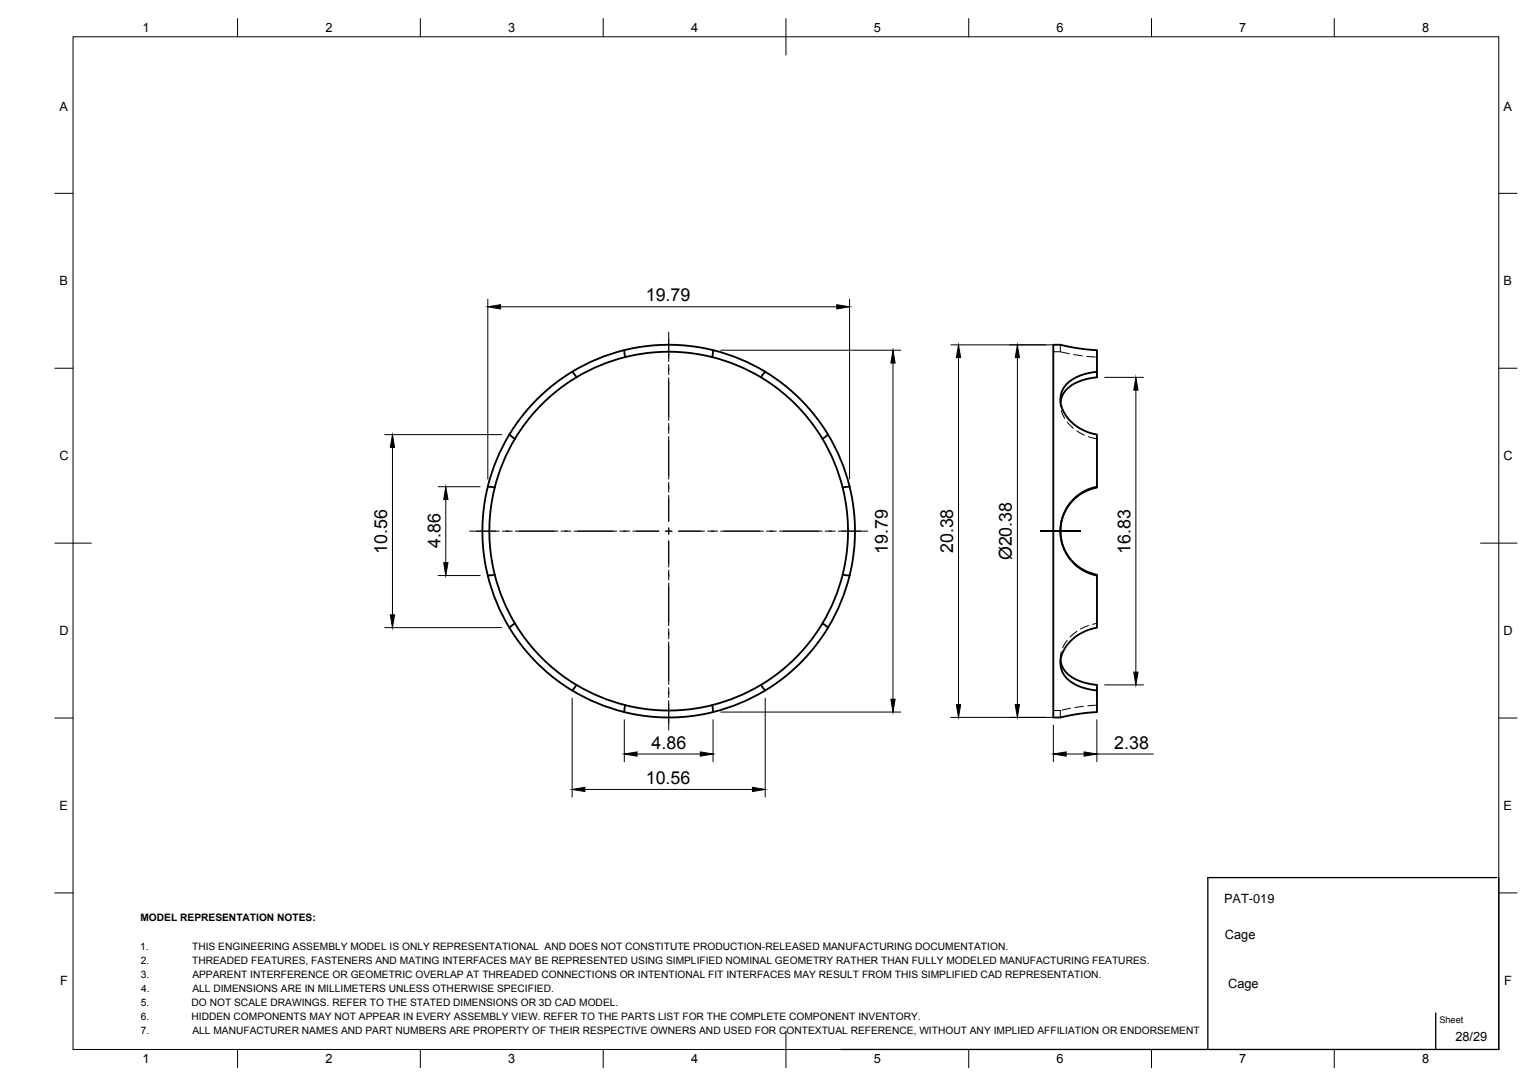
ISO-10303-21;
HEADER;
/* Generated by software containing ST-Developer
 * from STEP Tools, Inc. (www.steptools.com) 
 */

FILE_DESCRIPTION(
/* description */ ('Caster wheel assembly'),
/* implementation_level */ '2;1');

FILE_NAME(
/* name */ 'Cage.step',
/* time_stamp */ '2026-10-28T03:23:56-07:00',
/* author */ (''),
/* organization */ (''),
/* preprocessor_version */ 'ST-DEVELOPER v20.2',
/* originating_system */ 'Autodesk Translation Framework v15.17.0.0',
/* authorisation */ '');

FILE_SCHEMA (('AUTOMOTIVE_DESIGN { 1 0 10303 214 3 1 1 }'));
ENDSEC;

DATA;
#10=MECHANICAL_DESIGN_GEOMETRIC_PRESENTATION_REPRESENTATION('',(#249),#5385);
#11=B_SPLINE_CURVE_WITH_KNOTS('',3,(#4844,#4845,#4846,#4847,#4848,#4849,
#4850,#4851,#4852,#4853,#4854,#4855,#4856,#4857,#4858,#4859,#4860,#4861,
#4862,#4863,#4864,#4865),.UNSPECIFIED.,.F.,.F.,(4,2,2,2,2,2,2,2,2,2,4),
(0.0473477652366656,0.126350602536658,0.189525903804987,0.252701205073317,
0.313298422430275,0.373895639787233,0.434492857144191,0.495090074501149,
0.558265375769478,0.621440677037807,0.7004435143378),.UNSPECIFIED.);
#12=B_SPLINE_CURVE_WITH_KNOTS('',3,(#4869,#4870,#4871,#4872,#4873,#4874,
#4875,#4876,#4877,#4878,#4879,#4880,#4881,#4882,#4883,#4884,#4885,#4886,
#4887,#4888,#4889,#4890),.UNSPECIFIED.,.F.,.F.,(4,2,2,2,2,2,2,2,2,2,4),
(0.0464897534940957,0.0852567806515119,0.170513561303024,0.246687263103517,
0.308657850341199,0.370628437578881,0.432599024816563,0.494569612054245,
0.570743313854739,0.656000094506251,0.694767121663666),.UNSPECIFIED.);
#13=B_SPLINE_CURVE_WITH_KNOTS('',3,(#4896,#4897,#4898,#4899,#4900,#4901,
#4902,#4903,#4904,#4905,#4906,#4907,#4908,#4909,#4910,#4911,#4912,#4913,
#4914,#4915,#4916,#4917),.UNSPECIFIED.,.F.,.F.,(4,2,2,2,2,2,2,2,2,2,4),
(0.0464897534940957,0.0852567806515118,0.170513561303024,0.246687263103517,
0.308657850341199,0.370628437578881,0.432599024816563,0.494569612054245,
0.570743313854738,0.65600009450625,0.694767121663666),.UNSPECIFIED.);
#14=B_SPLINE_CURVE_WITH_KNOTS('',3,(#4921,#4922,#4923,#4924,#4925,#4926,
#4927,#4928,#4929,#4930,#4931,#4932,#4933,#4934,#4935,#4936,#4937,#4938,
#4939,#4940,#4941,#4942),.UNSPECIFIED.,.F.,.F.,(4,2,2,2,2,2,2,2,2,2,4),
(0.0464897534940957,0.0852567806515119,0.170513561303024,0.246687263103517,
0.308657850341199,0.370628437578881,0.432599024816563,0.494569612054245,
0.570743313854739,0.656000094506251,0.694767121663666),.UNSPECIFIED.);
#15=B_SPLINE_CURVE_WITH_KNOTS('',3,(#4946,#4947,#4948,#4949,#4950,#4951,
#4952,#4953,#4954,#4955,#4956,#4957),.UNSPECIFIED.,.F.,.F.,(4,2,2,2,2,4),
(0.0464897534940957,0.0852567806515119,0.170513561303024,0.246687263103517,
0.308657850341199,0.370628437578881),.UNSPECIFIED.);
#16=B_SPLINE_CURVE_WITH_KNOTS('',3,(#4962,#4963,#4964,#4965,#4966,#4967,
#4968,#4969,#4970,#4971,#4972,#4973),.UNSPECIFIED.,.F.,.F.,(4,2,2,2,2,4),
(0.370628437578881,0.432599024816563,0.494569612054245,0.570743313854738,
0.65600009450625,0.694767121663666),.UNSPECIFIED.);
#17=B_SPLINE_CURVE_WITH_KNOTS('',3,(#4977,#4978,#4979,#4980,#4981,#4982,
#4983,#4984,#4985,#4986,#4987,#4988,#4989,#4990,#4991,#4992,#4993,#4994,
#4995,#4996,#4997,#4998),.UNSPECIFIED.,.F.,.F.,(4,2,2,2,2,2,2,2,2,2,4),
(0.0464897534940957,0.0852567806515121,0.170513561303024,0.246687263103518,
0.308657850341199,0.370628437578881,0.432599024816563,0.494569612054245,
0.570743313854738,0.65600009450625,0.694767121663666),.UNSPECIFIED.);
#18=B_SPLINE_CURVE_WITH_KNOTS('',3,(#5002,#5003,#5004,#5005,#5006,#5007,
#5008,#5009,#5010,#5011,#5012,#5013,#5014,#5015,#5016,#5017,#5018,#5019,
#5020,#5021,#5022,#5023),.UNSPECIFIED.,.F.,.F.,(4,2,2,2,2,2,2,2,2,2,4),
(0.0464897534940957,0.0852567806515119,0.170513561303024,0.246687263103517,
0.308657850341199,0.370628437578881,0.432599024816563,0.494569612054245,
0.570743313854738,0.65600009450625,0.694767121663667),.UNSPECIFIED.);
#19=B_SPLINE_CURVE_WITH_KNOTS('',3,(#5027,#5028,#5029,#5030,#5031,#5032,
#5033,#5034,#5035,#5036,#5037,#5038,#5039,#5040,#5041,#5042,#5043,#5044,
#5045,#5046,#5047,#5048),.UNSPECIFIED.,.F.,.F.,(4,2,2,2,2,2,2,2,2,2,4),
(0.0464897534940957,0.0852567806515119,0.170513561303024,0.246687263103517,
0.308657850341199,0.370628437578881,0.432599024816563,0.494569612054245,
0.570743313854738,0.65600009450625,0.694767121663666),.UNSPECIFIED.);
#20=B_SPLINE_CURVE_WITH_KNOTS('',3,(#5052,#5053,#5054,#5055,#5056,#5057,
#5058,#5059,#5060,#5061,#5062,#5063,#5064,#5065,#5066,#5067,#5068,#5069,
#5070,#5071,#5072,#5073),.UNSPECIFIED.,.F.,.F.,(4,2,2,2,2,2,2,2,2,2,4),
(0.0464897534940957,0.0852567806515119,0.170513561303024,0.246687263103517,
0.308657850341199,0.370628437578881,0.432599024816563,0.494569612054245,
0.570743313854739,0.656000094506251,0.694767121663667),.UNSPECIFIED.);
#21=B_SPLINE_CURVE_WITH_KNOTS('',3,(#5081,#5082,#5083,#5084,#5085,#5086,
#5087,#5088,#5089,#5090,#5091,#5092,#5093,#5094,#5095,#5096,#5097,#5098,
#5099,#5100,#5101,#5102),.UNSPECIFIED.,.F.,.F.,(4,2,2,2,2,2,2,2,2,2,4),
(0.0473477652366656,0.126350602536658,0.189525903804987,0.252701205073316,
0.313298422430274,0.373895639787232,0.434492857144191,0.495090074501149,
0.558265375769478,0.621440677037807,0.7004435143378),.UNSPECIFIED.);
#22=B_SPLINE_CURVE_WITH_KNOTS('',3,(#5110,#5111,#5112,#5113,#5114,#5115,
#5116,#5117,#5118,#5119,#5120,#5121,#5122,#5123,#5124,#5125,#5126,#5127,
#5128,#5129,#5130,#5131),.UNSPECIFIED.,.F.,.F.,(4,2,2,2,2,2,2,2,2,2,4),
(0.0473477652366656,0.126350602536658,0.189525903804987,0.252701205073317,
0.313298422430275,0.373895639787233,0.434492857144191,0.495090074501149,
0.558265375769478,0.621440677037807,0.7004435143378),.UNSPECIFIED.);
#23=B_SPLINE_CURVE_WITH_KNOTS('',3,(#5140,#5141,#5142,#5143,#5144,#5145,
#5146,#5147,#5148,#5149,#5150,#5151),.UNSPECIFIED.,.F.,.F.,(4,2,2,2,2,4),
(0.0473477652366656,0.126350602536658,0.189525903804987,0.252701205073316,
0.313298422430275,0.373895639787233),.UNSPECIFIED.);
#24=B_SPLINE_CURVE_WITH_KNOTS('',3,(#5153,#5154,#5155,#5156,#5157,#5158,
#5159,#5160,#5161,#5162,#5163,#5164),.UNSPECIFIED.,.F.,.F.,(4,2,2,2,2,4),
(0.373895639787233,0.434492857144191,0.495090074501149,0.558265375769478,
0.621440677037807,0.7004435143378),.UNSPECIFIED.);
#25=B_SPLINE_CURVE_WITH_KNOTS('',3,(#5171,#5172,#5173,#5174,#5175,#5176,
#5177,#5178,#5179,#5180,#5181,#5182,#5183,#5184,#5185,#5186,#5187,#5188,
#5189,#5190,#5191,#5192),.UNSPECIFIED.,.F.,.F.,(4,2,2,2,2,2,2,2,2,2,4),
(0.0473477652366656,0.126350602536658,0.189525903804987,0.252701205073316,
0.313298422430275,0.373895639787233,0.434492857144191,0.495090074501149,
0.558265375769478,0.621440677037807,0.7004435143378),.UNSPECIFIED.);
#26=B_SPLINE_CURVE_WITH_KNOTS('',3,(#5200,#5201,#5202,#5203,#5204,#5205,
#5206,#5207,#5208,#5209,#5210,#5211,#5212,#5213,#5214,#5215,#5216,#5217,
#5218,#5219,#5220,#5221),.UNSPECIFIED.,.F.,.F.,(4,2,2,2,2,2,2,2,2,2,4),
(0.0473477652366656,0.126350602536658,0.189525903804987,0.252701205073317,
0.313298422430275,0.373895639787233,0.434492857144191,0.495090074501149,
0.558265375769478,0.621440677037807,0.7004435143378),.UNSPECIFIED.);
#27=B_SPLINE_CURVE_WITH_KNOTS('',3,(#5229,#5230,#5231,#5232,#5233,#5234,
#5235,#5236,#5237,#5238,#5239,#5240,#5241,#5242,#5243,#5244,#5245,#5246,
#5247,#5248,#5249,#5250),.UNSPECIFIED.,.F.,.F.,(4,2,2,2,2,2,2,2,2,2,4),
(0.0473477652366656,0.126350602536658,0.189525903804987,0.252701205073316,
0.313298422430275,0.373895639787233,0.434492857144191,0.495090074501149,
0.558265375769478,0.621440677037807,0.7004435143378),.UNSPECIFIED.);
#28=B_SPLINE_CURVE_WITH_KNOTS('',3,(#5259,#5260,#5261,#5262,#5263,#5264,
#5265,#5266,#5267,#5268,#5269,#5270,#5271,#5272,#5273,#5274,#5275,#5276,
#5277,#5278,#5279,#5280),.UNSPECIFIED.,.F.,.F.,(4,2,2,2,2,2,2,2,2,2,4),
(0.0473477652366656,0.126350602536658,0.189525903804987,0.252701205073317,
0.313298422430275,0.373895639787233,0.434492857144191,0.495090074501149,
0.558265375769478,0.621440677037807,0.7004435143378),.UNSPECIFIED.);
#37=SPHERICAL_SURFACE('',#3221,0.247676);
#38=SPHERICAL_SURFACE('',#3237,0.247676);
#39=SPHERICAL_SURFACE('',#3242,0.247676);
#40=SPHERICAL_SURFACE('',#3247,0.247676);
#41=SPHERICAL_SURFACE('',#3252,0.247676);
#42=SPHERICAL_SURFACE('',#3257,0.247676);
#43=SPHERICAL_SURFACE('',#3262,0.247676);
#44=SPHERICAL_SURFACE('',#3270,0.247676);
#198=SHAPE_REPRESENTATION_RELATIONSHIP('SRR','None',#5496,#220);
#220=ADVANCED_BREP_SHAPE_REPRESENTATION('',(#278),#5383);
#249=STYLED_ITEM('',(#5672),#278);
#278=MANIFOLD_SOLID_BREP('Continuous crown cage',#2677);
#328=FACE_BOUND('',#795,.T.);
#408=PLANE('',#3234);
#409=PLANE('',#3239);
#410=PLANE('',#3244);
#411=PLANE('',#3249);
#412=PLANE('',#3254);
#413=PLANE('',#3259);
#414=PLANE('',#3268);
#415=PLANE('',#3272);
#416=PLANE('',#3273);
#562=FACE_OUTER_BOUND('',#777,.T.);
#563=FACE_OUTER_BOUND('',#778,.T.);
#564=FACE_OUTER_BOUND('',#779,.T.);
#565=FACE_OUTER_BOUND('',#780,.T.);
#566=FACE_OUTER_BOUND('',#781,.T.);
#567=FACE_OUTER_BOUND('',#782,.T.);
#568=FACE_OUTER_BOUND('',#783,.T.);
#569=FACE_OUTER_BOUND('',#784,.T.);
#570=FACE_OUTER_BOUND('',#785,.T.);
#571=FACE_OUTER_BOUND('',#786,.T.);
#572=FACE_OUTER_BOUND('',#787,.T.);
#573=FACE_OUTER_BOUND('',#788,.T.);
#574=FACE_OUTER_BOUND('',#789,.T.);
#575=FACE_OUTER_BOUND('',#790,.T.);
#576=FACE_OUTER_BOUND('',#791,.T.);
#577=FACE_OUTER_BOUND('',#792,.T.);
#578=FACE_OUTER_BOUND('',#793,.T.);
#579=FACE_OUTER_BOUND('',#794,.T.);
#580=FACE_OUTER_BOUND('',#796,.T.);
#777=EDGE_LOOP('',(#2296,#2297,#2298,#2299));
#778=EDGE_LOOP('',(#2300,#2301,#2302,#2303,#2304,#2305,#2306,#2307,#2308,
#2309,#2310,#2311,#2312,#2313,#2314,#2315,#2316,#2317,#2318,#2319));
#779=EDGE_LOOP('',(#2320,#2321,#2322,#2323));
#780=EDGE_LOOP('',(#2324,#2325,#2326,#2327));
#781=EDGE_LOOP('',(#2328,#2329,#2330,#2331));
#782=EDGE_LOOP('',(#2332,#2333,#2334,#2335));
#783=EDGE_LOOP('',(#2336,#2337,#2338,#2339));
#784=EDGE_LOOP('',(#2340,#2341,#2342,#2343,#2344,#2345));
#785=EDGE_LOOP('',(#2346,#2347,#2348,#2349));
#786=EDGE_LOOP('',(#2350,#2351,#2352,#2353));
#787=EDGE_LOOP('',(#2354,#2355,#2356,#2357));
#788=EDGE_LOOP('',(#2358,#2359,#2360,#2361));
#789=EDGE_LOOP('',(#2362,#2363,#2364,#2365));
#790=EDGE_LOOP('',(#2366,#2367,#2368,#2369));
#791=EDGE_LOOP('',(#2370,#2371,#2372,#2373,#2374,#2375,#2376,#2377,#2378,
#2379,#2380,#2381,#2382,#2383,#2384,#2385,#2386,#2387,#2388,#2389));
#792=EDGE_LOOP('',(#2390,#2391,#2392,#2393));
#793=EDGE_LOOP('',(#2394,#2395,#2396,#2397));
#794=EDGE_LOOP('',(#2398));
#795=EDGE_LOOP('',(#2399));
#796=EDGE_LOOP('',(#2400,#2401,#2402,#2403));
#937=LINE('',#4959,#1071);
#938=LINE('',#5255,#1072);
#1071=VECTOR('',#4042,1.019052);
#1072=VECTOR('',#4119,0.980948);
#1194=CIRCLE('',#3222,0.243053047864041);
#1195=CIRCLE('',#3223,0.243053047864041);
#1196=CIRCLE('',#3225,1.019052);
#1197=CIRCLE('',#3226,1.019052);
#1198=CIRCLE('',#3227,1.019052);
#1199=CIRCLE('',#3228,1.019052);
#1200=CIRCLE('',#3229,1.019052);
#1201=CIRCLE('',#3230,1.019052);
#1202=CIRCLE('',#3231,1.019052);
#1203=CIRCLE('',#3232,1.019052);
#1204=CIRCLE('',#3233,1.019052);
#1205=CIRCLE('',#3235,0.980948);
#1206=CIRCLE('',#3236,0.243053047864041);
#1207=CIRCLE('',#3238,0.243053047864041);
#1208=CIRCLE('',#3240,0.980948);
#1209=CIRCLE('',#3241,0.243053047864041);
#1210=CIRCLE('',#3243,0.243053047864041);
#1211=CIRCLE('',#3245,0.980948);
#1212=CIRCLE('',#3246,0.243053047864041);
#1213=CIRCLE('',#3248,0.243053047864041);
#1214=CIRCLE('',#3250,0.980948);
#1215=CIRCLE('',#3251,0.243053047864041);
#1216=CIRCLE('',#3253,0.243053047864041);
#1217=CIRCLE('',#3255,0.980948);
#1218=CIRCLE('',#3256,0.243053047864041);
#1219=CIRCLE('',#3258,0.243053047864041);
#1220=CIRCLE('',#3260,0.980948);
#1221=CIRCLE('',#3261,0.243053047864041);
#1222=CIRCLE('',#3263,0.243053047864041);
#1223=CIRCLE('',#3265,0.980948);
#1224=CIRCLE('',#3266,0.980948);
#1225=CIRCLE('',#3267,0.980948);
#1226=CIRCLE('',#3269,0.243053047864041);
#1227=CIRCLE('',#3271,0.243053047864041);
#1415=VERTEX_POINT('',#4842);
#1416=VERTEX_POINT('',#4843);
#1417=VERTEX_POINT('',#4866);
#1418=VERTEX_POINT('',#4868);
#1419=VERTEX_POINT('',#4893);
#1420=VERTEX_POINT('',#4895);
#1421=VERTEX_POINT('',#4918);
#1422=VERTEX_POINT('',#4920);
#1423=VERTEX_POINT('',#4943);
#1424=VERTEX_POINT('',#4945);
#1425=VERTEX_POINT('',#4958);
#1426=VERTEX_POINT('',#4961);
#1427=VERTEX_POINT('',#4974);
#1428=VERTEX_POINT('',#4976);
#1429=VERTEX_POINT('',#4999);
#1430=VERTEX_POINT('',#5001);
#1431=VERTEX_POINT('',#5024);
#1432=VERTEX_POINT('',#5026);
#1433=VERTEX_POINT('',#5049);
#1434=VERTEX_POINT('',#5051);
#1435=VERTEX_POINT('',#5076);
#1436=VERTEX_POINT('',#5080);
#1437=VERTEX_POINT('',#5105);
#1438=VERTEX_POINT('',#5109);
#1439=VERTEX_POINT('',#5134);
#1440=VERTEX_POINT('',#5138);
#1441=VERTEX_POINT('',#5139);
#1442=VERTEX_POINT('',#5166);
#1443=VERTEX_POINT('',#5170);
#1444=VERTEX_POINT('',#5195);
#1445=VERTEX_POINT('',#5199);
#1446=VERTEX_POINT('',#5224);
#1447=VERTEX_POINT('',#5228);
#1448=VERTEX_POINT('',#5253);
#1449=VERTEX_POINT('',#5256);
#1450=VERTEX_POINT('',#5258);
#1716=EDGE_CURVE('',#1415,#1416,#11,.T.);
#1717=EDGE_CURVE('',#1417,#1415,#1194,.T.);
#1718=EDGE_CURVE('',#1418,#1417,#12,.T.);
#1719=EDGE_CURVE('',#1416,#1418,#1195,.T.);
#1720=EDGE_CURVE('',#1419,#1417,#1196,.T.);
#1721=EDGE_CURVE('',#1419,#1420,#13,.T.);
#1722=EDGE_CURVE('',#1421,#1420,#1197,.T.);
#1723=EDGE_CURVE('',#1421,#1422,#14,.T.);
#1724=EDGE_CURVE('',#1423,#1422,#1198,.T.);
#1725=EDGE_CURVE('',#1423,#1424,#15,.T.);
#1726=EDGE_CURVE('',#1424,#1425,#937,.T.);
#1727=EDGE_CURVE('',#1425,#1425,#1199,.T.);
#1728=EDGE_CURVE('',#1424,#1426,#16,.T.);
#1729=EDGE_CURVE('',#1427,#1426,#1200,.T.);
#1730=EDGE_CURVE('',#1427,#1428,#17,.T.);
#1731=EDGE_CURVE('',#1429,#1428,#1201,.T.);
#1732=EDGE_CURVE('',#1429,#1430,#18,.T.);
#1733=EDGE_CURVE('',#1431,#1430,#1202,.T.);
#1734=EDGE_CURVE('',#1431,#1432,#19,.T.);
#1735=EDGE_CURVE('',#1433,#1432,#1203,.T.);
#1736=EDGE_CURVE('',#1433,#1434,#20,.T.);
#1737=EDGE_CURVE('',#1418,#1434,#1204,.T.);
#1738=EDGE_CURVE('',#1415,#1435,#1205,.T.);
#1739=EDGE_CURVE('',#1435,#1419,#1206,.T.);
#1740=EDGE_CURVE('',#1436,#1435,#21,.T.);
#1741=EDGE_CURVE('',#1420,#1436,#1207,.T.);
#1742=EDGE_CURVE('',#1436,#1437,#1208,.T.);
#1743=EDGE_CURVE('',#1437,#1421,#1209,.T.);
#1744=EDGE_CURVE('',#1438,#1437,#22,.T.);
#1745=EDGE_CURVE('',#1422,#1438,#1210,.T.);
#1746=EDGE_CURVE('',#1438,#1439,#1211,.T.);
#1747=EDGE_CURVE('',#1439,#1423,#1212,.T.);
#1748=EDGE_CURVE('',#1440,#1441,#23,.T.);
#1749=EDGE_CURVE('',#1426,#1440,#1213,.T.);
#1750=EDGE_CURVE('',#1441,#1439,#24,.T.);
#1751=EDGE_CURVE('',#1440,#1442,#1214,.T.);
#1752=EDGE_CURVE('',#1442,#1427,#1215,.T.);
#1753=EDGE_CURVE('',#1443,#1442,#25,.T.);
#1754=EDGE_CURVE('',#1428,#1443,#1216,.T.);
#1755=EDGE_CURVE('',#1443,#1444,#1217,.T.);
#1756=EDGE_CURVE('',#1444,#1429,#1218,.T.);
#1757=EDGE_CURVE('',#1445,#1444,#26,.T.);
#1758=EDGE_CURVE('',#1430,#1445,#1219,.T.);
#1759=EDGE_CURVE('',#1445,#1446,#1220,.T.);
#1760=EDGE_CURVE('',#1446,#1431,#1221,.T.);
#1761=EDGE_CURVE('',#1447,#1446,#27,.T.);
#1762=EDGE_CURVE('',#1432,#1447,#1222,.T.);
#1763=EDGE_CURVE('',#1448,#1448,#1223,.T.);
#1764=EDGE_CURVE('',#1448,#1441,#938,.T.);
#1765=EDGE_CURVE('',#1449,#1416,#1224,.T.);
#1766=EDGE_CURVE('',#1449,#1450,#28,.T.);
#1767=EDGE_CURVE('',#1447,#1450,#1225,.T.);
#1768=EDGE_CURVE('',#1434,#1449,#1226,.T.);
#1769=EDGE_CURVE('',#1450,#1433,#1227,.T.);
#2296=ORIENTED_EDGE('',*,*,#1716,.F.);
#2297=ORIENTED_EDGE('',*,*,#1717,.F.);
#2298=ORIENTED_EDGE('',*,*,#1718,.F.);
#2299=ORIENTED_EDGE('',*,*,#1719,.F.);
#2300=ORIENTED_EDGE('',*,*,#1718,.T.);
#2301=ORIENTED_EDGE('',*,*,#1720,.F.);
#2302=ORIENTED_EDGE('',*,*,#1721,.T.);
#2303=ORIENTED_EDGE('',*,*,#1722,.F.);
#2304=ORIENTED_EDGE('',*,*,#1723,.T.);
#2305=ORIENTED_EDGE('',*,*,#1724,.F.);
#2306=ORIENTED_EDGE('',*,*,#1725,.T.);
#2307=ORIENTED_EDGE('',*,*,#1726,.T.);
#2308=ORIENTED_EDGE('',*,*,#1727,.F.);
#2309=ORIENTED_EDGE('',*,*,#1726,.F.);
#2310=ORIENTED_EDGE('',*,*,#1728,.T.);
#2311=ORIENTED_EDGE('',*,*,#1729,.F.);
#2312=ORIENTED_EDGE('',*,*,#1730,.T.);
#2313=ORIENTED_EDGE('',*,*,#1731,.F.);
#2314=ORIENTED_EDGE('',*,*,#1732,.T.);
#2315=ORIENTED_EDGE('',*,*,#1733,.F.);
#2316=ORIENTED_EDGE('',*,*,#1734,.T.);
#2317=ORIENTED_EDGE('',*,*,#1735,.F.);
#2318=ORIENTED_EDGE('',*,*,#1736,.T.);
#2319=ORIENTED_EDGE('',*,*,#1737,.F.);
#2320=ORIENTED_EDGE('',*,*,#1717,.T.);
#2321=ORIENTED_EDGE('',*,*,#1738,.T.);
#2322=ORIENTED_EDGE('',*,*,#1739,.T.);
#2323=ORIENTED_EDGE('',*,*,#1720,.T.);
#2324=ORIENTED_EDGE('',*,*,#1740,.F.);
#2325=ORIENTED_EDGE('',*,*,#1741,.F.);
#2326=ORIENTED_EDGE('',*,*,#1721,.F.);
#2327=ORIENTED_EDGE('',*,*,#1739,.F.);
#2328=ORIENTED_EDGE('',*,*,#1741,.T.);
#2329=ORIENTED_EDGE('',*,*,#1742,.T.);
#2330=ORIENTED_EDGE('',*,*,#1743,.T.);
#2331=ORIENTED_EDGE('',*,*,#1722,.T.);
#2332=ORIENTED_EDGE('',*,*,#1744,.F.);
#2333=ORIENTED_EDGE('',*,*,#1745,.F.);
#2334=ORIENTED_EDGE('',*,*,#1723,.F.);
#2335=ORIENTED_EDGE('',*,*,#1743,.F.);
#2336=ORIENTED_EDGE('',*,*,#1745,.T.);
#2337=ORIENTED_EDGE('',*,*,#1746,.T.);
#2338=ORIENTED_EDGE('',*,*,#1747,.T.);
#2339=ORIENTED_EDGE('',*,*,#1724,.T.);
#2340=ORIENTED_EDGE('',*,*,#1748,.F.);
#2341=ORIENTED_EDGE('',*,*,#1749,.F.);
#2342=ORIENTED_EDGE('',*,*,#1728,.F.);
#2343=ORIENTED_EDGE('',*,*,#1725,.F.);
#2344=ORIENTED_EDGE('',*,*,#1747,.F.);
#2345=ORIENTED_EDGE('',*,*,#1750,.F.);
#2346=ORIENTED_EDGE('',*,*,#1749,.T.);
#2347=ORIENTED_EDGE('',*,*,#1751,.T.);
#2348=ORIENTED_EDGE('',*,*,#1752,.T.);
#2349=ORIENTED_EDGE('',*,*,#1729,.T.);
#2350=ORIENTED_EDGE('',*,*,#1753,.F.);
#2351=ORIENTED_EDGE('',*,*,#1754,.F.);
#2352=ORIENTED_EDGE('',*,*,#1730,.F.);
#2353=ORIENTED_EDGE('',*,*,#1752,.F.);
#2354=ORIENTED_EDGE('',*,*,#1754,.T.);
#2355=ORIENTED_EDGE('',*,*,#1755,.T.);
#2356=ORIENTED_EDGE('',*,*,#1756,.T.);
#2357=ORIENTED_EDGE('',*,*,#1731,.T.);
#2358=ORIENTED_EDGE('',*,*,#1757,.F.);
#2359=ORIENTED_EDGE('',*,*,#1758,.F.);
#2360=ORIENTED_EDGE('',*,*,#1732,.F.);
#2361=ORIENTED_EDGE('',*,*,#1756,.F.);
#2362=ORIENTED_EDGE('',*,*,#1758,.T.);
#2363=ORIENTED_EDGE('',*,*,#1759,.T.);
#2364=ORIENTED_EDGE('',*,*,#1760,.T.);
#2365=ORIENTED_EDGE('',*,*,#1733,.T.);
#2366=ORIENTED_EDGE('',*,*,#1734,.F.);
#2367=ORIENTED_EDGE('',*,*,#1760,.F.);
#2368=ORIENTED_EDGE('',*,*,#1761,.F.);
#2369=ORIENTED_EDGE('',*,*,#1762,.F.);
#2370=ORIENTED_EDGE('',*,*,#1763,.F.);
#2371=ORIENTED_EDGE('',*,*,#1764,.T.);
#2372=ORIENTED_EDGE('',*,*,#1750,.T.);
#2373=ORIENTED_EDGE('',*,*,#1746,.F.);
#2374=ORIENTED_EDGE('',*,*,#1744,.T.);
#2375=ORIENTED_EDGE('',*,*,#1742,.F.);
#2376=ORIENTED_EDGE('',*,*,#1740,.T.);
#2377=ORIENTED_EDGE('',*,*,#1738,.F.);
#2378=ORIENTED_EDGE('',*,*,#1716,.T.);
#2379=ORIENTED_EDGE('',*,*,#1765,.F.);
#2380=ORIENTED_EDGE('',*,*,#1766,.T.);
#2381=ORIENTED_EDGE('',*,*,#1767,.F.);
#2382=ORIENTED_EDGE('',*,*,#1761,.T.);
#2383=ORIENTED_EDGE('',*,*,#1759,.F.);
#2384=ORIENTED_EDGE('',*,*,#1757,.T.);
#2385=ORIENTED_EDGE('',*,*,#1755,.F.);
#2386=ORIENTED_EDGE('',*,*,#1753,.T.);
#2387=ORIENTED_EDGE('',*,*,#1751,.F.);
#2388=ORIENTED_EDGE('',*,*,#1748,.T.);
#2389=ORIENTED_EDGE('',*,*,#1764,.F.);
#2390=ORIENTED_EDGE('',*,*,#1719,.T.);
#2391=ORIENTED_EDGE('',*,*,#1737,.T.);
#2392=ORIENTED_EDGE('',*,*,#1768,.T.);
#2393=ORIENTED_EDGE('',*,*,#1765,.T.);
#2394=ORIENTED_EDGE('',*,*,#1736,.F.);
#2395=ORIENTED_EDGE('',*,*,#1769,.F.);
#2396=ORIENTED_EDGE('',*,*,#1766,.F.);
#2397=ORIENTED_EDGE('',*,*,#1768,.F.);
#2398=ORIENTED_EDGE('',*,*,#1727,.T.);
#2399=ORIENTED_EDGE('',*,*,#1763,.T.);
#2400=ORIENTED_EDGE('',*,*,#1762,.T.);
#2401=ORIENTED_EDGE('',*,*,#1767,.T.);
#2402=ORIENTED_EDGE('',*,*,#1769,.T.);
#2403=ORIENTED_EDGE('',*,*,#1735,.T.);
#2475=CYLINDRICAL_SURFACE('',#3224,1.019052);
#2476=CYLINDRICAL_SURFACE('',#3264,0.980948);
#2622=ADVANCED_FACE('',(#562),#37,.F.);
#2623=ADVANCED_FACE('',(#563),#2475,.T.);
#2624=ADVANCED_FACE('',(#564),#408,.T.);
#2625=ADVANCED_FACE('',(#565),#38,.F.);
#2626=ADVANCED_FACE('',(#566),#409,.T.);
#2627=ADVANCED_FACE('',(#567),#39,.F.);
#2628=ADVANCED_FACE('',(#568),#410,.T.);
#2629=ADVANCED_FACE('',(#569),#40,.F.);
#2630=ADVANCED_FACE('',(#570),#411,.T.);
#2631=ADVANCED_FACE('',(#571),#41,.F.);
#2632=ADVANCED_FACE('',(#572),#412,.T.);
#2633=ADVANCED_FACE('',(#573),#42,.F.);
#2634=ADVANCED_FACE('',(#574),#413,.T.);
#2635=ADVANCED_FACE('',(#575),#43,.F.);
#2636=ADVANCED_FACE('',(#576),#2476,.F.);
#2637=ADVANCED_FACE('',(#577),#414,.T.);
#2638=ADVANCED_FACE('',(#578),#44,.F.);
#2639=ADVANCED_FACE('',(#579,#328),#415,.T.);
#2640=ADVANCED_FACE('',(#580),#416,.T.);
#2677=CLOSED_SHELL('',(#2622,#2623,#2624,#2625,#2626,#2627,#2628,#2629,
#2630,#2631,#2632,#2633,#2634,#2635,#2636,#2637,#2638,#2639,#2640));
#3220=AXIS2_PLACEMENT_3D('',#4840,#4026,#4027);
#3221=AXIS2_PLACEMENT_3D('',#4841,#4028,#4029);
#3222=AXIS2_PLACEMENT_3D('',#4867,#4030,#4031);
#3223=AXIS2_PLACEMENT_3D('',#4891,#4032,#4033);
#3224=AXIS2_PLACEMENT_3D('',#4892,#4034,#4035);
#3225=AXIS2_PLACEMENT_3D('',#4894,#4036,#4037);
#3226=AXIS2_PLACEMENT_3D('',#4919,#4038,#4039);
#3227=AXIS2_PLACEMENT_3D('',#4944,#4040,#4041);
#3228=AXIS2_PLACEMENT_3D('',#4960,#4043,#4044);
#3229=AXIS2_PLACEMENT_3D('',#4975,#4045,#4046);
#3230=AXIS2_PLACEMENT_3D('',#5000,#4047,#4048);
#3231=AXIS2_PLACEMENT_3D('',#5025,#4049,#4050);
#3232=AXIS2_PLACEMENT_3D('',#5050,#4051,#4052);
#3233=AXIS2_PLACEMENT_3D('',#5074,#4053,#4054);
#3234=AXIS2_PLACEMENT_3D('',#5075,#4055,#4056);
#3235=AXIS2_PLACEMENT_3D('',#5077,#4057,#4058);
#3236=AXIS2_PLACEMENT_3D('',#5078,#4059,#4060);
#3237=AXIS2_PLACEMENT_3D('',#5079,#4061,#4062);
#3238=AXIS2_PLACEMENT_3D('',#5103,#4063,#4064);
#3239=AXIS2_PLACEMENT_3D('',#5104,#4065,#4066);
#3240=AXIS2_PLACEMENT_3D('',#5106,#4067,#4068);
#3241=AXIS2_PLACEMENT_3D('',#5107,#4069,#4070);
#3242=AXIS2_PLACEMENT_3D('',#5108,#4071,#4072);
#3243=AXIS2_PLACEMENT_3D('',#5132,#4073,#4074);
#3244=AXIS2_PLACEMENT_3D('',#5133,#4075,#4076);
#3245=AXIS2_PLACEMENT_3D('',#5135,#4077,#4078);
#3246=AXIS2_PLACEMENT_3D('',#5136,#4079,#4080);
#3247=AXIS2_PLACEMENT_3D('',#5137,#4081,#4082);
#3248=AXIS2_PLACEMENT_3D('',#5152,#4083,#4084);
#3249=AXIS2_PLACEMENT_3D('',#5165,#4085,#4086);
#3250=AXIS2_PLACEMENT_3D('',#5167,#4087,#4088);
#3251=AXIS2_PLACEMENT_3D('',#5168,#4089,#4090);
#3252=AXIS2_PLACEMENT_3D('',#5169,#4091,#4092);
#3253=AXIS2_PLACEMENT_3D('',#5193,#4093,#4094);
#3254=AXIS2_PLACEMENT_3D('',#5194,#4095,#4096);
#3255=AXIS2_PLACEMENT_3D('',#5196,#4097,#4098);
#3256=AXIS2_PLACEMENT_3D('',#5197,#4099,#4100);
#3257=AXIS2_PLACEMENT_3D('',#5198,#4101,#4102);
#3258=AXIS2_PLACEMENT_3D('',#5222,#4103,#4104);
#3259=AXIS2_PLACEMENT_3D('',#5223,#4105,#4106);
#3260=AXIS2_PLACEMENT_3D('',#5225,#4107,#4108);
#3261=AXIS2_PLACEMENT_3D('',#5226,#4109,#4110);
#3262=AXIS2_PLACEMENT_3D('',#5227,#4111,#4112);
#3263=AXIS2_PLACEMENT_3D('',#5251,#4113,#4114);
#3264=AXIS2_PLACEMENT_3D('',#5252,#4115,#4116);
#3265=AXIS2_PLACEMENT_3D('',#5254,#4117,#4118);
#3266=AXIS2_PLACEMENT_3D('',#5257,#4120,#4121);
#3267=AXIS2_PLACEMENT_3D('',#5281,#4122,#4123);
#3268=AXIS2_PLACEMENT_3D('',#5282,#4124,#4125);
#3269=AXIS2_PLACEMENT_3D('',#5283,#4126,#4127);
#3270=AXIS2_PLACEMENT_3D('',#5284,#4128,#4129);
#3271=AXIS2_PLACEMENT_3D('',#5285,#4130,#4131);
#3272=AXIS2_PLACEMENT_3D('',#5286,#4132,#4133);
#3273=AXIS2_PLACEMENT_3D('',#5287,#4134,#4135);
#4026=DIRECTION('axis',(0.,0.,1.));
#4027=DIRECTION('refdir',(1.,0.,0.));
#4028=DIRECTION('center_axis',(0.,0.,1.));
#4029=DIRECTION('ref_axis',(1.,0.,0.));
#4030=DIRECTION('center_axis',(0.,-1.,0.));
#4031=DIRECTION('ref_axis',(0.,0.,-1.));
#4032=DIRECTION('center_axis',(0.,-1.,0.));
#4033=DIRECTION('ref_axis',(0.,0.,-1.));
#4034=DIRECTION('center_axis',(0.,1.,0.));
#4035=DIRECTION('ref_axis',(1.,0.,0.));
#4036=DIRECTION('center_axis',(0.,1.,0.));
#4037=DIRECTION('ref_axis',(1.,0.,0.));
#4038=DIRECTION('center_axis',(0.,1.,0.));
#4039=DIRECTION('ref_axis',(1.,0.,0.));
#4040=DIRECTION('center_axis',(0.,1.,0.));
#4041=DIRECTION('ref_axis',(1.,0.,0.));
#4042=DIRECTION('',(0.,-1.,0.));
#4043=DIRECTION('center_axis',(0.,-1.,0.));
#4044=DIRECTION('ref_axis',(1.,0.,0.));
#4045=DIRECTION('center_axis',(0.,1.,0.));
#4046=DIRECTION('ref_axis',(1.,0.,0.));
#4047=DIRECTION('center_axis',(0.,1.,0.));
#4048=DIRECTION('ref_axis',(1.,0.,0.));
#4049=DIRECTION('center_axis',(0.,1.,0.));
#4050=DIRECTION('ref_axis',(1.,0.,0.));
#4051=DIRECTION('center_axis',(0.,1.,0.));
#4052=DIRECTION('ref_axis',(1.,0.,0.));
#4053=DIRECTION('center_axis',(0.,1.,0.));
#4054=DIRECTION('ref_axis',(1.,0.,0.));
#4055=DIRECTION('center_axis',(0.,1.,0.));
#4056=DIRECTION('ref_axis',(1.,0.,0.));
#4057=DIRECTION('center_axis',(0.,-1.,0.));
#4058=DIRECTION('ref_axis',(1.,0.,0.));
#4059=DIRECTION('center_axis',(0.,-1.,0.));
#4060=DIRECTION('ref_axis',(0.,0.,-1.));
#4061=DIRECTION('center_axis',(6.12323399573677E-17,0.,1.));
#4062=DIRECTION('ref_axis',(1.,0.,0.));
#4063=DIRECTION('center_axis',(0.,-1.,0.));
#4064=DIRECTION('ref_axis',(0.,0.,-1.));
#4065=DIRECTION('center_axis',(0.,1.,0.));
#4066=DIRECTION('ref_axis',(1.,0.,0.));
#4067=DIRECTION('center_axis',(0.,-1.,0.));
#4068=DIRECTION('ref_axis',(1.,0.,0.));
#4069=DIRECTION('center_axis',(0.,-1.,0.));
#4070=DIRECTION('ref_axis',(0.,0.,-1.));
#4071=DIRECTION('center_axis',(0.,0.,1.));
#4072=DIRECTION('ref_axis',(1.,0.,0.));
#4073=DIRECTION('center_axis',(0.,-1.,0.));
#4074=DIRECTION('ref_axis',(0.,0.,-1.));
#4075=DIRECTION('center_axis',(0.,1.,0.));
#4076=DIRECTION('ref_axis',(1.,0.,0.));
#4077=DIRECTION('center_axis',(0.,-1.,0.));
#4078=DIRECTION('ref_axis',(1.,0.,0.));
#4079=DIRECTION('center_axis',(0.,-1.,0.));
#4080=DIRECTION('ref_axis',(0.,0.,-1.));
#4081=DIRECTION('center_axis',(0.,0.,1.));
#4082=DIRECTION('ref_axis',(1.,0.,0.));
#4083=DIRECTION('center_axis',(0.,-1.,0.));
#4084=DIRECTION('ref_axis',(0.,0.,-1.));
#4085=DIRECTION('center_axis',(0.,1.,0.));
#4086=DIRECTION('ref_axis',(1.,0.,0.));
#4087=DIRECTION('center_axis',(0.,-1.,0.));
#4088=DIRECTION('ref_axis',(1.,0.,0.));
#4089=DIRECTION('center_axis',(0.,-1.,0.));
#4090=DIRECTION('ref_axis',(0.,0.,-1.));
#4091=DIRECTION('center_axis',(0.,0.,1.));
#4092=DIRECTION('ref_axis',(1.,0.,0.));
#4093=DIRECTION('center_axis',(0.,-1.,0.));
#4094=DIRECTION('ref_axis',(0.,0.,-1.));
#4095=DIRECTION('center_axis',(0.,1.,0.));
#4096=DIRECTION('ref_axis',(1.,0.,0.));
#4097=DIRECTION('center_axis',(0.,-1.,0.));
#4098=DIRECTION('ref_axis',(1.,0.,0.));
#4099=DIRECTION('center_axis',(0.,-1.,0.));
#4100=DIRECTION('ref_axis',(0.,0.,-1.));
#4101=DIRECTION('center_axis',(6.12323399573676E-17,0.,1.));
#4102=DIRECTION('ref_axis',(1.,0.,0.));
#4103=DIRECTION('center_axis',(0.,-1.,0.));
#4104=DIRECTION('ref_axis',(0.,0.,-1.));
#4105=DIRECTION('center_axis',(0.,1.,0.));
#4106=DIRECTION('ref_axis',(1.,0.,0.));
#4107=DIRECTION('center_axis',(0.,-1.,0.));
#4108=DIRECTION('ref_axis',(1.,0.,0.));
#4109=DIRECTION('center_axis',(0.,-1.,0.));
#4110=DIRECTION('ref_axis',(0.,0.,-1.));
#4111=DIRECTION('center_axis',(0.,0.,1.));
#4112=DIRECTION('ref_axis',(1.,0.,0.));
#4113=DIRECTION('center_axis',(0.,-1.,0.));
#4114=DIRECTION('ref_axis',(0.,0.,-1.));
#4115=DIRECTION('center_axis',(0.,1.,0.));
#4116=DIRECTION('ref_axis',(1.,0.,0.));
#4117=DIRECTION('center_axis',(0.,1.,0.));
#4118=DIRECTION('ref_axis',(1.,0.,0.));
#4119=DIRECTION('',(0.,1.,0.));
#4120=DIRECTION('center_axis',(0.,-1.,0.));
#4121=DIRECTION('ref_axis',(1.,0.,0.));
#4122=DIRECTION('center_axis',(0.,-1.,0.));
#4123=DIRECTION('ref_axis',(1.,0.,0.));
#4124=DIRECTION('center_axis',(0.,1.,0.));
#4125=DIRECTION('ref_axis',(1.,0.,0.));
#4126=DIRECTION('center_axis',(0.,-1.,0.));
#4127=DIRECTION('ref_axis',(0.,0.,-1.));
#4128=DIRECTION('center_axis',(0.,0.,1.));
#4129=DIRECTION('ref_axis',(1.,0.,0.));
#4130=DIRECTION('center_axis',(0.,-1.,0.));
#4131=DIRECTION('ref_axis',(0.,0.,-1.));
#4132=DIRECTION('center_axis',(0.,-1.,0.));
#4133=DIRECTION('ref_axis',(-1.,0.,0.));
#4134=DIRECTION('center_axis',(0.,1.,0.));
#4135=DIRECTION('ref_axis',(1.,0.,0.));
#4840=CARTESIAN_POINT('',(0.,0.,0.));
#4841=CARTESIAN_POINT('Origin',(0.707106781186547,0.,0.707106781186548));
#4842=CARTESIAN_POINT('',(0.504455939115715,-0.04763,0.841298510752802));
#4843=CARTESIAN_POINT('',(0.841298510752802,-0.04763,0.504455939115715));
#4844=CARTESIAN_POINT('Ctrl Pts',(0.504455939115715,-0.04763,0.841298510752802));
#4845=CARTESIAN_POINT('Ctrl Pts',(0.508899795931835,-0.0740444353928835,
0.838633903678357));
#4846=CARTESIAN_POINT('Ctrl Pts',(0.517157748491652,-0.0999305678883309,
0.833661031856294));
#4847=CARTESIAN_POINT('Ctrl Pts',(0.537715343527944,-0.142345102874864,
0.820511285096538));
#4848=CARTESIAN_POINT('Ctrl Pts',(0.548874290046456,-0.159766064500479,
0.813159949759));
#4849=CARTESIAN_POINT('Ctrl Pts',(0.573915184558107,-0.190326085855194,
0.795684265985089));
#4850=CARTESIAN_POINT('Ctrl Pts',(0.587792702767295,-0.203463743702801,
0.78555112003688));
#4851=CARTESIAN_POINT('Ctrl Pts',(0.615966552324775,-0.224161999508995,
0.763642258217233));
#4852=CARTESIAN_POINT('Ctrl Pts',(0.631684198665438,-0.232861760990032,
0.750785745543687));
#4853=CARTESIAN_POINT('Ctrl Pts',(0.663382628119203,-0.244251601209411,
0.722929908501543));
#4854=CARTESIAN_POINT('Ctrl Pts',(0.679352081686668,-0.246942143572133,
0.707917883896095));
#4855=CARTESIAN_POINT('Ctrl Pts',(0.707917883896095,-0.246942143572133,
0.679352081686668));
#4856=CARTESIAN_POINT('Ctrl Pts',(0.722929908501543,-0.244251601209411,
0.663382628119203));
#4857=CARTESIAN_POINT('Ctrl Pts',(0.750785745543687,-0.232861760990032,
0.631684198665439));
#4858=CARTESIAN_POINT('Ctrl Pts',(0.763642258217232,-0.224161999508995,
0.615966552324775));
#4859=CARTESIAN_POINT('Ctrl Pts',(0.78555112003688,-0.203463743702801,0.587792702767295));
#4860=CARTESIAN_POINT('Ctrl Pts',(0.795684265985088,-0.190326085855194,
0.573915184558108));
#4861=CARTESIAN_POINT('Ctrl Pts',(0.813159949759,-0.15976606450048,0.548874290046456));
#4862=CARTESIAN_POINT('Ctrl Pts',(0.820511285096538,-0.142345102874864,
0.537715343527944));
#4863=CARTESIAN_POINT('Ctrl Pts',(0.833661031856294,-0.099930567888331,
0.517157748491653));
#4864=CARTESIAN_POINT('Ctrl Pts',(0.838633903678357,-0.0740444353928835,
0.508899795931835));
#4865=CARTESIAN_POINT('Ctrl Pts',(0.841298510752801,-0.0476299999999999,
0.504455939115715));
#4866=CARTESIAN_POINT('',(0.528110872004958,-0.04763,0.871530771444223));
#4867=CARTESIAN_POINT('Origin',(0.707106781186547,-0.04763,0.707106781186548));
#4868=CARTESIAN_POINT('',(0.871530771444223,-0.04763,0.528110872004959));
#4869=CARTESIAN_POINT('Ctrl Pts',(0.871530771444223,-0.0476300000000001,
0.528110872004958));
#4870=CARTESIAN_POINT('Ctrl Pts',(0.87014664509073,-0.0609922781173483,
0.530395067942936));
#4871=CARTESIAN_POINT('Ctrl Pts',(0.868149331745851,-0.0742967091364493,
0.533674141594226));
#4872=CARTESIAN_POINT('Ctrl Pts',(0.85981294420286,-0.115492077056649,0.54708917182331));
#4873=CARTESIAN_POINT('Ctrl Pts',(0.850993704737257,-0.141695629206859,
0.560922177770136));
#4874=CARTESIAN_POINT('Ctrl Pts',(0.830754510485543,-0.181890537957859,
0.590422647829571));
#4875=CARTESIAN_POINT('Ctrl Pts',(0.816896541396381,-0.201072148666545,
0.609616703125488));
#4876=CARTESIAN_POINT('Ctrl Pts',(0.792310597819928,-0.223955109275652,
0.641117951819998));
#4877=CARTESIAN_POINT('Ctrl Pts',(0.779109323683612,-0.232742381310829,
0.657208095763053));
#4878=CARTESIAN_POINT('Ctrl Pts',(0.750552691816206,-0.244234834628584,
0.68964083160521));
#4879=CARTESIAN_POINT('Ctrl Pts',(0.735185187071673,-0.246942143572133,
0.705971972091755));
#4880=CARTESIAN_POINT('Ctrl Pts',(0.705971972091754,-0.246942143572133,
0.735185187071673));
#4881=CARTESIAN_POINT('Ctrl Pts',(0.689640831605209,-0.244234834628584,
0.750552691816206));
#4882=CARTESIAN_POINT('Ctrl Pts',(0.657208095763052,-0.232742381310829,
0.779109323683612));
#4883=CARTESIAN_POINT('Ctrl Pts',(0.641117951819998,-0.223955109275652,
0.792310597819928));
#4884=CARTESIAN_POINT('Ctrl Pts',(0.609616703125487,-0.201072148666545,
0.816896541396382));
#4885=CARTESIAN_POINT('Ctrl Pts',(0.590422647829571,-0.181890537957858,
0.830754510485544));
#4886=CARTESIAN_POINT('Ctrl Pts',(0.560922177770135,-0.141695629206858,
0.850993704737257));
#4887=CARTESIAN_POINT('Ctrl Pts',(0.547089171823309,-0.115492077056649,
0.859812944202861));
#4888=CARTESIAN_POINT('Ctrl Pts',(0.533674141594226,-0.0742967091364491,
0.868149331745852));
#4889=CARTESIAN_POINT('Ctrl Pts',(0.530395067942936,-0.0609922781173483,
0.870146645090731));
#4890=CARTESIAN_POINT('Ctrl Pts',(0.528110872004958,-0.0476300000000001,
0.871530771444223));
#4891=CARTESIAN_POINT('Origin',(0.707106781186547,-0.04763,0.707106781186548));
#4892=CARTESIAN_POINT('Origin',(0.,-0.166705,0.));
#4893=CARTESIAN_POINT('',(0.242834539687906,-0.04763,0.989696097314));
#4894=CARTESIAN_POINT('Origin',(0.,-0.04763,0.));
#4895=CARTESIAN_POINT('',(-0.242834539687907,-0.04763,0.989696097314));
#4896=CARTESIAN_POINT('Ctrl Pts',(0.242834539687906,-0.04763,0.989696097314));
#4897=CARTESIAN_POINT('Ctrl Pts',(0.24024064412003,-0.0609922781173483,
0.990332542620729));
#4898=CARTESIAN_POINT('Ctrl Pts',(0.236509675094874,-0.0742967091364492,
0.991238884025248));
#4899=CARTESIAN_POINT('Ctrl Pts',(0.221129100087819,-0.115492077056649,
0.994830026707808));
#4900=CARTESIAN_POINT('Ctrl Pts',(0.205111543747588,-0.141695629206859,
0.998375294985966));
#4901=CARTESIAN_POINT('Ctrl Pts',(0.169940289819232,-0.181890537957859,
1.00492400591205));
#4902=CARTESIAN_POINT('Ctrl Pts',(0.1465689792446,-0.201072148666545,1.00869718865384));
#4903=CARTESIAN_POINT('Ctrl Pts',(0.106909345252087,-0.223955109275652,
1.01358704779679));
#4904=CARTESIAN_POINT('Ctrl Pts',(0.0861971848975941,-0.232742381310829,
1.0156297872271));
#4905=CARTESIAN_POINT('Ctrl Pts',(0.0430711894098822,-0.244234834628584,
1.01837060663223));
#4906=CARTESIAN_POINT('Ctrl Pts',(0.0206568624125605,-0.246942143572133,
1.019052));
#4907=CARTESIAN_POINT('Ctrl Pts',(-0.0206568624125608,-0.246942143572133,
1.019052));
#4908=CARTESIAN_POINT('Ctrl Pts',(-0.0430711894098825,-0.244234834628584,
1.01837060663223));
#4909=CARTESIAN_POINT('Ctrl Pts',(-0.0861971848975943,-0.232742381310829,
1.0156297872271));
#4910=CARTESIAN_POINT('Ctrl Pts',(-0.106909345252088,-0.223955109275652,
1.01358704779679));
#4911=CARTESIAN_POINT('Ctrl Pts',(-0.1465689792446,-0.201072148666545,1.00869718865384));
#4912=CARTESIAN_POINT('Ctrl Pts',(-0.169940289819232,-0.181890537957859,
1.00492400591205));
#4913=CARTESIAN_POINT('Ctrl Pts',(-0.205111543747588,-0.141695629206859,
0.998375294985966));
#4914=CARTESIAN_POINT('Ctrl Pts',(-0.221129100087819,-0.115492077056649,
0.994830026707808));
#4915=CARTESIAN_POINT('Ctrl Pts',(-0.236509675094875,-0.0742967091364493,
0.991238884025248));
#4916=CARTESIAN_POINT('Ctrl Pts',(-0.24024064412003,-0.0609922781173483,
0.990332542620729));
#4917=CARTESIAN_POINT('Ctrl Pts',(-0.242834539687907,-0.04763,0.989696097314));
#4918=CARTESIAN_POINT('',(-0.528110872004959,-0.04763,0.871530771444223));
#4919=CARTESIAN_POINT('Origin',(0.,-0.04763,0.));
#4920=CARTESIAN_POINT('',(-0.871530771444223,-0.04763,0.528110872004958));
#4921=CARTESIAN_POINT('Ctrl Pts',(-0.528110872004958,-0.0476300000000001,
0.871530771444223));
#4922=CARTESIAN_POINT('Ctrl Pts',(-0.530395067942936,-0.0609922781173484,
0.87014664509073));
#4923=CARTESIAN_POINT('Ctrl Pts',(-0.533674141594226,-0.0742967091364493,
0.868149331745851));
#4924=CARTESIAN_POINT('Ctrl Pts',(-0.54708917182331,-0.115492077056649,
0.85981294420286));
#4925=CARTESIAN_POINT('Ctrl Pts',(-0.560922177770136,-0.141695629206859,
0.850993704737257));
#4926=CARTESIAN_POINT('Ctrl Pts',(-0.590422647829571,-0.181890537957859,
0.830754510485543));
#4927=CARTESIAN_POINT('Ctrl Pts',(-0.609616703125488,-0.201072148666545,
0.816896541396381));
#4928=CARTESIAN_POINT('Ctrl Pts',(-0.641117951819998,-0.223955109275652,
0.792310597819928));
#4929=CARTESIAN_POINT('Ctrl Pts',(-0.657208095763053,-0.232742381310829,
0.779109323683611));
#4930=CARTESIAN_POINT('Ctrl Pts',(-0.68964083160521,-0.244234834628584,
0.750552691816205));
#4931=CARTESIAN_POINT('Ctrl Pts',(-0.705971972091755,-0.246942143572133,
0.735185187071673));
#4932=CARTESIAN_POINT('Ctrl Pts',(-0.735185187071673,-0.246942143572133,
0.705971972091754));
#4933=CARTESIAN_POINT('Ctrl Pts',(-0.750552691816206,-0.244234834628584,
0.689640831605209));
#4934=CARTESIAN_POINT('Ctrl Pts',(-0.779109323683612,-0.232742381310829,
0.657208095763052));
#4935=CARTESIAN_POINT('Ctrl Pts',(-0.792310597819928,-0.223955109275652,
0.641117951819998));
#4936=CARTESIAN_POINT('Ctrl Pts',(-0.816896541396382,-0.201072148666545,
0.609616703125487));
#4937=CARTESIAN_POINT('Ctrl Pts',(-0.830754510485544,-0.181890537957858,
0.590422647829571));
#4938=CARTESIAN_POINT('Ctrl Pts',(-0.850993704737257,-0.141695629206858,
0.560922177770135));
#4939=CARTESIAN_POINT('Ctrl Pts',(-0.859812944202861,-0.115492077056649,
0.547089171823309));
#4940=CARTESIAN_POINT('Ctrl Pts',(-0.868149331745852,-0.0742967091364491,
0.533674141594226));
#4941=CARTESIAN_POINT('Ctrl Pts',(-0.870146645090731,-0.0609922781173483,
0.530395067942936));
#4942=CARTESIAN_POINT('Ctrl Pts',(-0.871530771444223,-0.04763,0.528110872004958));
#4943=CARTESIAN_POINT('',(-0.989696097314,-0.04763,0.242834539687906));
#4944=CARTESIAN_POINT('Origin',(0.,-0.04763,0.));
#4945=CARTESIAN_POINT('',(-1.019052,-0.246942143572133,1.248489836334E-16));
#4946=CARTESIAN_POINT('Ctrl Pts',(-0.989696097314,-0.04763,0.242834539687906));
#4947=CARTESIAN_POINT('Ctrl Pts',(-0.990332542620729,-0.0609922781173483,
0.24024064412003));
#4948=CARTESIAN_POINT('Ctrl Pts',(-0.991238884025248,-0.0742967091364492,
0.236509675094874));
#4949=CARTESIAN_POINT('Ctrl Pts',(-0.994830026707808,-0.115492077056649,
0.221129100087819));
#4950=CARTESIAN_POINT('Ctrl Pts',(-0.998375294985966,-0.141695629206859,
0.205111543747588));
#4951=CARTESIAN_POINT('Ctrl Pts',(-1.00492400591205,-0.181890537957859,
0.169940289819232));
#4952=CARTESIAN_POINT('Ctrl Pts',(-1.00869718865384,-0.201072148666545,
0.1465689792446));
#4953=CARTESIAN_POINT('Ctrl Pts',(-1.01358704779679,-0.223955109275652,
0.106909345252088));
#4954=CARTESIAN_POINT('Ctrl Pts',(-1.0156297872271,-0.232742381310829,0.0861971848975944));
#4955=CARTESIAN_POINT('Ctrl Pts',(-1.01837060663223,-0.244234834628584,
0.0430711894098825));
#4956=CARTESIAN_POINT('Ctrl Pts',(-1.019052,-0.246942143572133,0.0206568624125608));
#4957=CARTESIAN_POINT('Ctrl Pts',(-1.019052,-0.246942143572133,1.2490009027033E-16));
#4958=CARTESIAN_POINT('',(-1.019052,-0.28578,1.24797876996471E-16));
#4959=CARTESIAN_POINT('',(-1.019052,-0.166705,1.24797876996471E-16));
#4960=CARTESIAN_POINT('Origin',(0.,-0.28578,0.));
#4961=CARTESIAN_POINT('',(-0.989696097314,-0.04763,-0.242834539687906));
#4962=CARTESIAN_POINT('Ctrl Pts',(-1.019052,-0.246942143572133,1.2490009027033E-16));
#4963=CARTESIAN_POINT('Ctrl Pts',(-1.019052,-0.246942143572133,-0.0206568624125605));
#4964=CARTESIAN_POINT('Ctrl Pts',(-1.01837060663223,-0.244234834628584,
-0.0430711894098822));
#4965=CARTESIAN_POINT('Ctrl Pts',(-1.0156297872271,-0.232742381310829,-0.0861971848975941));
#4966=CARTESIAN_POINT('Ctrl Pts',(-1.01358704779679,-0.223955109275652,
-0.106909345252087));
#4967=CARTESIAN_POINT('Ctrl Pts',(-1.00869718865384,-0.201072148666546,
-0.1465689792446));
#4968=CARTESIAN_POINT('Ctrl Pts',(-1.00492400591205,-0.181890537957859,
-0.169940289819232));
#4969=CARTESIAN_POINT('Ctrl Pts',(-0.998375294985966,-0.141695629206859,
-0.205111543747588));
#4970=CARTESIAN_POINT('Ctrl Pts',(-0.994830026707808,-0.11549207705665,
-0.221129100087819));
#4971=CARTESIAN_POINT('Ctrl Pts',(-0.991238884025248,-0.0742967091364495,
-0.236509675094874));
#4972=CARTESIAN_POINT('Ctrl Pts',(-0.990332542620729,-0.0609922781173484,
-0.24024064412003));
#4973=CARTESIAN_POINT('Ctrl Pts',(-0.989696097314,-0.0476300000000001,-0.242834539687907));
#4974=CARTESIAN_POINT('',(-0.871530771444223,-0.04763,-0.528110872004958));
#4975=CARTESIAN_POINT('Origin',(0.,-0.04763,0.));
#4976=CARTESIAN_POINT('',(-0.528110872004958,-0.04763,-0.871530771444223));
#4977=CARTESIAN_POINT('Ctrl Pts',(-0.871530771444223,-0.0476300000000001,
-0.528110872004958));
#4978=CARTESIAN_POINT('Ctrl Pts',(-0.87014664509073,-0.0609922781173484,
-0.530395067942936));
#4979=CARTESIAN_POINT('Ctrl Pts',(-0.868149331745851,-0.0742967091364494,
-0.533674141594226));
#4980=CARTESIAN_POINT('Ctrl Pts',(-0.85981294420286,-0.115492077056649,
-0.54708917182331));
#4981=CARTESIAN_POINT('Ctrl Pts',(-0.850993704737257,-0.141695629206859,
-0.560922177770136));
#4982=CARTESIAN_POINT('Ctrl Pts',(-0.830754510485543,-0.181890537957859,
-0.590422647829571));
#4983=CARTESIAN_POINT('Ctrl Pts',(-0.816896541396381,-0.201072148666546,
-0.609616703125488));
#4984=CARTESIAN_POINT('Ctrl Pts',(-0.792310597819928,-0.223955109275652,
-0.641117951819999));
#4985=CARTESIAN_POINT('Ctrl Pts',(-0.779109323683611,-0.232742381310829,
-0.657208095763053));
#4986=CARTESIAN_POINT('Ctrl Pts',(-0.750552691816205,-0.244234834628584,
-0.68964083160521));
#4987=CARTESIAN_POINT('Ctrl Pts',(-0.735185187071673,-0.246942143572133,
-0.705971972091755));
#4988=CARTESIAN_POINT('Ctrl Pts',(-0.705971972091754,-0.246942143572133,
-0.735185187071673));
#4989=CARTESIAN_POINT('Ctrl Pts',(-0.68964083160521,-0.244234834628584,
-0.750552691816206));
#4990=CARTESIAN_POINT('Ctrl Pts',(-0.657208095763052,-0.232742381310829,
-0.779109323683612));
#4991=CARTESIAN_POINT('Ctrl Pts',(-0.641117951819998,-0.223955109275652,
-0.792310597819928));
#4992=CARTESIAN_POINT('Ctrl Pts',(-0.609616703125488,-0.201072148666545,
-0.816896541396381));
#4993=CARTESIAN_POINT('Ctrl Pts',(-0.590422647829571,-0.181890537957859,
-0.830754510485543));
#4994=CARTESIAN_POINT('Ctrl Pts',(-0.560922177770136,-0.141695629206859,
-0.850993704737257));
#4995=CARTESIAN_POINT('Ctrl Pts',(-0.54708917182331,-0.115492077056649,
-0.85981294420286));
#4996=CARTESIAN_POINT('Ctrl Pts',(-0.533674141594226,-0.0742967091364494,
-0.868149331745852));
#4997=CARTESIAN_POINT('Ctrl Pts',(-0.530395067942936,-0.0609922781173484,
-0.870146645090731));
#4998=CARTESIAN_POINT('Ctrl Pts',(-0.528110872004958,-0.0476300000000001,
-0.871530771444223));
#4999=CARTESIAN_POINT('',(-0.242834539687906,-0.04763,-0.989696097314));
#5000=CARTESIAN_POINT('Origin',(0.,-0.04763,0.));
#5001=CARTESIAN_POINT('',(0.242834539687906,-0.04763,-0.989696097314));
#5002=CARTESIAN_POINT('Ctrl Pts',(-0.242834539687907,-0.04763,-0.989696097314));
#5003=CARTESIAN_POINT('Ctrl Pts',(-0.24024064412003,-0.0609922781173483,
-0.990332542620729));
#5004=CARTESIAN_POINT('Ctrl Pts',(-0.236509675094874,-0.0742967091364493,
-0.991238884025248));
#5005=CARTESIAN_POINT('Ctrl Pts',(-0.221129100087819,-0.115492077056649,
-0.994830026707808));
#5006=CARTESIAN_POINT('Ctrl Pts',(-0.205111543747588,-0.141695629206859,
-0.998375294985966));
#5007=CARTESIAN_POINT('Ctrl Pts',(-0.169940289819232,-0.181890537957859,
-1.00492400591205));
#5008=CARTESIAN_POINT('Ctrl Pts',(-0.1465689792446,-0.201072148666545,-1.00869718865384));
#5009=CARTESIAN_POINT('Ctrl Pts',(-0.106909345252087,-0.223955109275652,
-1.01358704779679));
#5010=CARTESIAN_POINT('Ctrl Pts',(-0.0861971848975942,-0.232742381310829,
-1.0156297872271));
#5011=CARTESIAN_POINT('Ctrl Pts',(-0.0430711894098823,-0.244234834628584,
-1.01837060663223));
#5012=CARTESIAN_POINT('Ctrl Pts',(-0.0206568624125606,-0.246942143572133,
-1.019052));
#5013=CARTESIAN_POINT('Ctrl Pts',(0.0206568624125607,-0.246942143572133,
-1.019052));
#5014=CARTESIAN_POINT('Ctrl Pts',(0.0430711894098824,-0.244234834628584,
-1.01837060663223));
#5015=CARTESIAN_POINT('Ctrl Pts',(0.0861971848975943,-0.232742381310829,
-1.0156297872271));
#5016=CARTESIAN_POINT('Ctrl Pts',(0.106909345252088,-0.223955109275652,
-1.01358704779679));
#5017=CARTESIAN_POINT('Ctrl Pts',(0.1465689792446,-0.201072148666545,-1.00869718865384));
#5018=CARTESIAN_POINT('Ctrl Pts',(0.169940289819232,-0.181890537957859,
-1.00492400591205));
#5019=CARTESIAN_POINT('Ctrl Pts',(0.205111543747588,-0.141695629206859,
-0.998375294985966));
#5020=CARTESIAN_POINT('Ctrl Pts',(0.221129100087819,-0.115492077056649,
-0.994830026707808));
#5021=CARTESIAN_POINT('Ctrl Pts',(0.236509675094874,-0.0742967091364493,
-0.991238884025248));
#5022=CARTESIAN_POINT('Ctrl Pts',(0.24024064412003,-0.0609922781173484,
-0.990332542620729));
#5023=CARTESIAN_POINT('Ctrl Pts',(0.242834539687907,-0.04763,-0.989696097314));
#5024=CARTESIAN_POINT('',(0.528110872004958,-0.04763,-0.871530771444223));
#5025=CARTESIAN_POINT('Origin',(0.,-0.04763,0.));
#5026=CARTESIAN_POINT('',(0.871530771444223,-0.04763,-0.528110872004958));
#5027=CARTESIAN_POINT('Ctrl Pts',(0.528110872004958,-0.0476300000000001,
-0.871530771444223));
#5028=CARTESIAN_POINT('Ctrl Pts',(0.530395067942936,-0.0609922781173484,
-0.870146645090731));
#5029=CARTESIAN_POINT('Ctrl Pts',(0.533674141594226,-0.0742967091364493,
-0.868149331745851));
#5030=CARTESIAN_POINT('Ctrl Pts',(0.54708917182331,-0.115492077056649,-0.85981294420286));
#5031=CARTESIAN_POINT('Ctrl Pts',(0.560922177770136,-0.141695629206859,
-0.850993704737257));
#5032=CARTESIAN_POINT('Ctrl Pts',(0.590422647829571,-0.181890537957859,
-0.830754510485543));
#5033=CARTESIAN_POINT('Ctrl Pts',(0.609616703125488,-0.201072148666545,
-0.816896541396381));
#5034=CARTESIAN_POINT('Ctrl Pts',(0.641117951819998,-0.223955109275652,
-0.792310597819928));
#5035=CARTESIAN_POINT('Ctrl Pts',(0.657208095763053,-0.232742381310829,
-0.779109323683612));
#5036=CARTESIAN_POINT('Ctrl Pts',(0.68964083160521,-0.244234834628584,-0.750552691816206));
#5037=CARTESIAN_POINT('Ctrl Pts',(0.705971972091755,-0.246942143572133,
-0.735185187071673));
#5038=CARTESIAN_POINT('Ctrl Pts',(0.735185187071673,-0.246942143572133,
-0.705971972091754));
#5039=CARTESIAN_POINT('Ctrl Pts',(0.750552691816206,-0.244234834628584,
-0.68964083160521));
#5040=CARTESIAN_POINT('Ctrl Pts',(0.779109323683612,-0.232742381310829,
-0.657208095763053));
#5041=CARTESIAN_POINT('Ctrl Pts',(0.792310597819928,-0.223955109275652,
-0.641117951819998));
#5042=CARTESIAN_POINT('Ctrl Pts',(0.816896541396381,-0.201072148666545,
-0.609616703125488));
#5043=CARTESIAN_POINT('Ctrl Pts',(0.830754510485543,-0.181890537957859,
-0.590422647829571));
#5044=CARTESIAN_POINT('Ctrl Pts',(0.850993704737257,-0.141695629206859,
-0.560922177770136));
#5045=CARTESIAN_POINT('Ctrl Pts',(0.85981294420286,-0.115492077056649,-0.54708917182331));
#5046=CARTESIAN_POINT('Ctrl Pts',(0.868149331745851,-0.0742967091364493,
-0.533674141594226));
#5047=CARTESIAN_POINT('Ctrl Pts',(0.870146645090731,-0.0609922781173484,
-0.530395067942936));
#5048=CARTESIAN_POINT('Ctrl Pts',(0.871530771444223,-0.0476300000000001,
-0.528110872004958));
#5049=CARTESIAN_POINT('',(0.989696097314,-0.04763,-0.242834539687906));
#5050=CARTESIAN_POINT('Origin',(0.,-0.04763,0.));
#5051=CARTESIAN_POINT('',(0.989696097314,-0.04763,0.242834539687906));
#5052=CARTESIAN_POINT('Ctrl Pts',(0.989696097314,-0.04763,-0.242834539687907));
#5053=CARTESIAN_POINT('Ctrl Pts',(0.990332542620729,-0.0609922781173483,
-0.24024064412003));
#5054=CARTESIAN_POINT('Ctrl Pts',(0.991238884025248,-0.0742967091364493,
-0.236509675094874));
#5055=CARTESIAN_POINT('Ctrl Pts',(0.994830026707808,-0.115492077056649,
-0.221129100087819));
#5056=CARTESIAN_POINT('Ctrl Pts',(0.998375294985966,-0.141695629206859,
-0.205111543747588));
#5057=CARTESIAN_POINT('Ctrl Pts',(1.00492400591205,-0.181890537957859,-0.169940289819232));
#5058=CARTESIAN_POINT('Ctrl Pts',(1.00869718865384,-0.201072148666545,-0.1465689792446));
#5059=CARTESIAN_POINT('Ctrl Pts',(1.01358704779679,-0.223955109275652,-0.106909345252087));
#5060=CARTESIAN_POINT('Ctrl Pts',(1.0156297872271,-0.232742381310829,-0.0861971848975942));
#5061=CARTESIAN_POINT('Ctrl Pts',(1.01837060663223,-0.244234834628584,-0.0430711894098823));
#5062=CARTESIAN_POINT('Ctrl Pts',(1.019052,-0.246942143572133,-0.0206568624125607));
#5063=CARTESIAN_POINT('Ctrl Pts',(1.019052,-0.246942143572133,0.0206568624125607));
#5064=CARTESIAN_POINT('Ctrl Pts',(1.01837060663223,-0.244234834628584,0.0430711894098823));
#5065=CARTESIAN_POINT('Ctrl Pts',(1.0156297872271,-0.232742381310829,0.0861971848975942));
#5066=CARTESIAN_POINT('Ctrl Pts',(1.01358704779679,-0.223955109275652,0.106909345252087));
#5067=CARTESIAN_POINT('Ctrl Pts',(1.00869718865384,-0.201072148666545,0.1465689792446));
#5068=CARTESIAN_POINT('Ctrl Pts',(1.00492400591205,-0.181890537957859,0.169940289819232));
#5069=CARTESIAN_POINT('Ctrl Pts',(0.998375294985966,-0.141695629206859,
0.205111543747588));
#5070=CARTESIAN_POINT('Ctrl Pts',(0.994830026707808,-0.115492077056649,
0.221129100087819));
#5071=CARTESIAN_POINT('Ctrl Pts',(0.991238884025248,-0.0742967091364492,
0.236509675094874));
#5072=CARTESIAN_POINT('Ctrl Pts',(0.990332542620729,-0.0609922781173483,
0.24024064412003));
#5073=CARTESIAN_POINT('Ctrl Pts',(0.989696097314,-0.04763,0.242834539687907));
#5074=CARTESIAN_POINT('Origin',(0.,-0.04763,0.));
#5075=CARTESIAN_POINT('Origin',(0.,-0.04763,0.));
#5076=CARTESIAN_POINT('',(0.238183666596899,-0.04763,0.951592097314));
#5077=CARTESIAN_POINT('Origin',(0.,-0.04763,0.));
#5078=CARTESIAN_POINT('Origin',(-1.94289029309402E-16,-0.04763,1.));
#5079=CARTESIAN_POINT('Origin',(-1.94289029309402E-16,0.,1.));
#5080=CARTESIAN_POINT('',(-0.2381836665969,-0.04763,0.951592097314));
#5081=CARTESIAN_POINT('Ctrl Pts',(-0.238183666596899,-0.0476299999999999,
0.951592097314));
#5082=CARTESIAN_POINT('Ctrl Pts',(-0.233157223576062,-0.0740444353928835,
0.952850216871763));
#5083=CARTESIAN_POINT('Ctrl Pts',(-0.223801617934946,-0.0999305678883309,
0.955173119738174));
#5084=CARTESIAN_POINT('Ctrl Pts',(-0.199966927975188,-0.142345102874864,
0.960411259488514));
#5085=CARTESIAN_POINT('Ctrl Pts',(-0.1868781821531,-0.159766064500479,0.963103647174702));
#5086=CARTESIAN_POINT('Ctrl Pts',(-0.15681442133453,-0.190326085855194,
0.968453058988463));
#5087=CARTESIAN_POINT('Ctrl Pts',(-0.139836317888043,-0.203463743702801,
0.971100730005489));
#5088=CARTESIAN_POINT('Ctrl Pts',(-0.104422493053067,-0.224161999508995,
0.975530745318961));
#5089=CARTESIAN_POINT('Ctrl Pts',(-0.0842175114474176,-0.232861760990032,
0.977553872336861));
#5090=CARTESIAN_POINT('Ctrl Pts',(-0.0421062857595701,-0.244251601209411,
0.980270995488453));
#5091=CARTESIAN_POINT('Ctrl Pts',(-0.0201990724523197,-0.246942143572133,
0.980948));
#5092=CARTESIAN_POINT('Ctrl Pts',(0.020199072452319,-0.246942143572133,
0.980948));
#5093=CARTESIAN_POINT('Ctrl Pts',(0.0421062857595694,-0.244251601209411,
0.980270995488454));
#5094=CARTESIAN_POINT('Ctrl Pts',(0.0842175114474169,-0.232861760990032,
0.977553872336861));
#5095=CARTESIAN_POINT('Ctrl Pts',(0.104422493053067,-0.224161999508995,
0.975530745318961));
#5096=CARTESIAN_POINT('Ctrl Pts',(0.139836317888042,-0.203463743702801,
0.971100730005489));
#5097=CARTESIAN_POINT('Ctrl Pts',(0.15681442133453,-0.190326085855194,0.968453058988463));
#5098=CARTESIAN_POINT('Ctrl Pts',(0.1868781821531,-0.15976606450048,0.963103647174702));
#5099=CARTESIAN_POINT('Ctrl Pts',(0.199966927975188,-0.142345102874864,
0.960411259488514));
#5100=CARTESIAN_POINT('Ctrl Pts',(0.223801617934945,-0.0999305678883309,
0.955173119738174));
#5101=CARTESIAN_POINT('Ctrl Pts',(0.233157223576061,-0.0740444353928835,
0.952850216871763));
#5102=CARTESIAN_POINT('Ctrl Pts',(0.238183666596899,-0.0476299999999999,
0.951592097314));
#5103=CARTESIAN_POINT('Origin',(-1.94289029309402E-16,-0.04763,1.));
#5104=CARTESIAN_POINT('Origin',(0.,-0.04763,0.));
#5105=CARTESIAN_POINT('',(-0.504455939115715,-0.04763,0.841298510752802));
#5106=CARTESIAN_POINT('Origin',(0.,-0.04763,0.));
#5107=CARTESIAN_POINT('Origin',(-0.707106781186548,-0.04763,0.707106781186547));
#5108=CARTESIAN_POINT('Origin',(-0.707106781186548,0.,0.707106781186547));
#5109=CARTESIAN_POINT('',(-0.841298510752802,-0.04763,0.504455939115715));
#5110=CARTESIAN_POINT('Ctrl Pts',(-0.841298510752802,-0.04763,0.504455939115715));
#5111=CARTESIAN_POINT('Ctrl Pts',(-0.838633903678357,-0.0740444353928835,
0.508899795931835));
#5112=CARTESIAN_POINT('Ctrl Pts',(-0.833661031856294,-0.0999305678883309,
0.517157748491652));
#5113=CARTESIAN_POINT('Ctrl Pts',(-0.820511285096538,-0.142345102874864,
0.537715343527944));
#5114=CARTESIAN_POINT('Ctrl Pts',(-0.813159949759,-0.159766064500479,0.548874290046456));
#5115=CARTESIAN_POINT('Ctrl Pts',(-0.795684265985089,-0.190326085855194,
0.573915184558107));
#5116=CARTESIAN_POINT('Ctrl Pts',(-0.78555112003688,-0.203463743702801,
0.587792702767295));
#5117=CARTESIAN_POINT('Ctrl Pts',(-0.763642258217233,-0.224161999508995,
0.615966552324775));
#5118=CARTESIAN_POINT('Ctrl Pts',(-0.750785745543687,-0.232861760990032,
0.631684198665438));
#5119=CARTESIAN_POINT('Ctrl Pts',(-0.722929908501543,-0.244251601209411,
0.663382628119203));
#5120=CARTESIAN_POINT('Ctrl Pts',(-0.707917883896095,-0.246942143572133,
0.679352081686668));
#5121=CARTESIAN_POINT('Ctrl Pts',(-0.679352081686668,-0.246942143572133,
0.707917883896095));
#5122=CARTESIAN_POINT('Ctrl Pts',(-0.663382628119203,-0.244251601209411,
0.722929908501544));
#5123=CARTESIAN_POINT('Ctrl Pts',(-0.631684198665438,-0.232861760990031,
0.750785745543687));
#5124=CARTESIAN_POINT('Ctrl Pts',(-0.615966552324775,-0.224161999508995,
0.763642258217233));
#5125=CARTESIAN_POINT('Ctrl Pts',(-0.587792702767295,-0.203463743702801,
0.78555112003688));
#5126=CARTESIAN_POINT('Ctrl Pts',(-0.573915184558107,-0.190326085855194,
0.795684265985088));
#5127=CARTESIAN_POINT('Ctrl Pts',(-0.548874290046456,-0.159766064500479,
0.813159949759));
#5128=CARTESIAN_POINT('Ctrl Pts',(-0.537715343527944,-0.142345102874864,
0.820511285096538));
#5129=CARTESIAN_POINT('Ctrl Pts',(-0.517157748491652,-0.0999305678883309,
0.833661031856294));
#5130=CARTESIAN_POINT('Ctrl Pts',(-0.508899795931835,-0.0740444353928835,
0.838633903678357));
#5131=CARTESIAN_POINT('Ctrl Pts',(-0.504455939115716,-0.04763,0.841298510752801));
#5132=CARTESIAN_POINT('Origin',(-0.707106781186548,-0.04763,0.707106781186547));
#5133=CARTESIAN_POINT('Origin',(0.,-0.04763,0.));
#5134=CARTESIAN_POINT('',(-0.951592097314,-0.04763,0.238183666596899));
#5135=CARTESIAN_POINT('Origin',(0.,-0.04763,0.));
#5136=CARTESIAN_POINT('Origin',(-1.,-0.04763,-1.11022302462516E-16));
#5137=CARTESIAN_POINT('Origin',(-1.,0.,-1.11022302462516E-16));
#5138=CARTESIAN_POINT('',(-0.951592097314,-0.04763,-0.2381836665969));
#5139=CARTESIAN_POINT('',(-0.980948,-0.246942143572133,1.08514323328844E-18));
#5140=CARTESIAN_POINT('Ctrl Pts',(-0.951592097314,-0.04763,-0.238183666596899));
#5141=CARTESIAN_POINT('Ctrl Pts',(-0.952850216871763,-0.0740444353928835,
-0.233157223576062));
#5142=CARTESIAN_POINT('Ctrl Pts',(-0.955173119738174,-0.0999305678883309,
-0.223801617934946));
#5143=CARTESIAN_POINT('Ctrl Pts',(-0.960411259488514,-0.142345102874864,
-0.199966927975188));
#5144=CARTESIAN_POINT('Ctrl Pts',(-0.963103647174702,-0.159766064500479,
-0.1868781821531));
#5145=CARTESIAN_POINT('Ctrl Pts',(-0.968453058988463,-0.190326085855194,
-0.15681442133453));
#5146=CARTESIAN_POINT('Ctrl Pts',(-0.971100730005489,-0.203463743702801,
-0.139836317888043));
#5147=CARTESIAN_POINT('Ctrl Pts',(-0.975530745318961,-0.224161999508995,
-0.104422493053067));
#5148=CARTESIAN_POINT('Ctrl Pts',(-0.977553872336861,-0.232861760990032,
-0.0842175114474175));
#5149=CARTESIAN_POINT('Ctrl Pts',(-0.980270995488453,-0.244251601209411,
-0.0421062857595699));
#5150=CARTESIAN_POINT('Ctrl Pts',(-0.980948,-0.246942143572133,-0.0201990724523195));
#5151=CARTESIAN_POINT('Ctrl Pts',(-0.980948,-0.246942143572133,-1.17961196366423E-16));
#5152=CARTESIAN_POINT('Origin',(-1.,-0.04763,-1.11022302462516E-16));
#5153=CARTESIAN_POINT('Ctrl Pts',(-0.980948,-0.246942143572133,-1.17961196366423E-16));
#5154=CARTESIAN_POINT('Ctrl Pts',(-0.980948,-0.246942143572133,0.0201990724523192));
#5155=CARTESIAN_POINT('Ctrl Pts',(-0.980270995488453,-0.244251601209411,
0.0421062857595695));
#5156=CARTESIAN_POINT('Ctrl Pts',(-0.977553872336861,-0.232861760990032,
0.0842175114474169));
#5157=CARTESIAN_POINT('Ctrl Pts',(-0.975530745318961,-0.224161999508995,
0.104422493053066));
#5158=CARTESIAN_POINT('Ctrl Pts',(-0.971100730005489,-0.203463743702801,
0.139836317888042));
#5159=CARTESIAN_POINT('Ctrl Pts',(-0.968453058988463,-0.190326085855194,
0.15681442133453));
#5160=CARTESIAN_POINT('Ctrl Pts',(-0.963103647174702,-0.15976606450048,
0.1868781821531));
#5161=CARTESIAN_POINT('Ctrl Pts',(-0.960411259488514,-0.142345102874864,
0.199966927975188));
#5162=CARTESIAN_POINT('Ctrl Pts',(-0.955173119738174,-0.099930567888331,
0.223801617934945));
#5163=CARTESIAN_POINT('Ctrl Pts',(-0.952850216871763,-0.0740444353928835,
0.233157223576061));
#5164=CARTESIAN_POINT('Ctrl Pts',(-0.951592097314,-0.04763,0.238183666596899));
#5165=CARTESIAN_POINT('Origin',(0.,-0.04763,0.));
#5166=CARTESIAN_POINT('',(-0.841298510752802,-0.04763,-0.504455939115715));
#5167=CARTESIAN_POINT('Origin',(0.,-0.04763,0.));
#5168=CARTESIAN_POINT('Origin',(-0.707106781186547,-0.04763,-0.707106781186548));
#5169=CARTESIAN_POINT('Origin',(-0.707106781186547,0.,-0.707106781186548));
#5170=CARTESIAN_POINT('',(-0.504455939115715,-0.04763,-0.841298510752802));
#5171=CARTESIAN_POINT('Ctrl Pts',(-0.504455939115715,-0.04763,-0.841298510752802));
#5172=CARTESIAN_POINT('Ctrl Pts',(-0.508899795931835,-0.0740444353928835,
-0.838633903678357));
#5173=CARTESIAN_POINT('Ctrl Pts',(-0.517157748491652,-0.0999305678883309,
-0.833661031856294));
#5174=CARTESIAN_POINT('Ctrl Pts',(-0.537715343527944,-0.142345102874864,
-0.820511285096538));
#5175=CARTESIAN_POINT('Ctrl Pts',(-0.548874290046456,-0.159766064500479,
-0.813159949759));
#5176=CARTESIAN_POINT('Ctrl Pts',(-0.573915184558107,-0.190326085855194,
-0.795684265985089));
#5177=CARTESIAN_POINT('Ctrl Pts',(-0.587792702767295,-0.203463743702801,
-0.78555112003688));
#5178=CARTESIAN_POINT('Ctrl Pts',(-0.615966552324775,-0.224161999508995,
-0.763642258217233));
#5179=CARTESIAN_POINT('Ctrl Pts',(-0.631684198665438,-0.232861760990032,
-0.750785745543687));
#5180=CARTESIAN_POINT('Ctrl Pts',(-0.663382628119203,-0.244251601209411,
-0.722929908501543));
#5181=CARTESIAN_POINT('Ctrl Pts',(-0.679352081686668,-0.246942143572133,
-0.707917883896095));
#5182=CARTESIAN_POINT('Ctrl Pts',(-0.707917883896095,-0.246942143572133,
-0.679352081686668));
#5183=CARTESIAN_POINT('Ctrl Pts',(-0.722929908501543,-0.244251601209411,
-0.663382628119203));
#5184=CARTESIAN_POINT('Ctrl Pts',(-0.750785745543687,-0.232861760990032,
-0.631684198665439));
#5185=CARTESIAN_POINT('Ctrl Pts',(-0.763642258217232,-0.224161999508995,
-0.615966552324775));
#5186=CARTESIAN_POINT('Ctrl Pts',(-0.78555112003688,-0.203463743702801,
-0.587792702767295));
#5187=CARTESIAN_POINT('Ctrl Pts',(-0.795684265985088,-0.190326085855194,
-0.573915184558107));
#5188=CARTESIAN_POINT('Ctrl Pts',(-0.813159949759,-0.15976606450048,-0.548874290046456));
#5189=CARTESIAN_POINT('Ctrl Pts',(-0.820511285096538,-0.142345102874864,
-0.537715343527944));
#5190=CARTESIAN_POINT('Ctrl Pts',(-0.833661031856294,-0.0999305678883311,
-0.517157748491652));
#5191=CARTESIAN_POINT('Ctrl Pts',(-0.838633903678357,-0.0740444353928836,
-0.508899795931835));
#5192=CARTESIAN_POINT('Ctrl Pts',(-0.841298510752801,-0.04763,-0.504455939115715));
#5193=CARTESIAN_POINT('Origin',(-0.707106781186547,-0.04763,-0.707106781186548));
#5194=CARTESIAN_POINT('Origin',(0.,-0.04763,0.));
#5195=CARTESIAN_POINT('',(-0.238183666596899,-0.04763,-0.951592097314));
#5196=CARTESIAN_POINT('Origin',(0.,-0.04763,0.));
#5197=CARTESIAN_POINT('Origin',(5.55111512312578E-17,-0.04763,-1.));
#5198=CARTESIAN_POINT('Origin',(5.55111512312578E-17,0.,-1.));
#5199=CARTESIAN_POINT('',(0.238183666596899,-0.04763,-0.951592097314));
#5200=CARTESIAN_POINT('Ctrl Pts',(0.238183666596899,-0.04763,-0.951592097314));
#5201=CARTESIAN_POINT('Ctrl Pts',(0.233157223576062,-0.0740444353928835,
-0.952850216871763));
#5202=CARTESIAN_POINT('Ctrl Pts',(0.223801617934946,-0.099930567888331,
-0.955173119738174));
#5203=CARTESIAN_POINT('Ctrl Pts',(0.199966927975188,-0.142345102874864,
-0.960411259488514));
#5204=CARTESIAN_POINT('Ctrl Pts',(0.1868781821531,-0.15976606450048,-0.963103647174702));
#5205=CARTESIAN_POINT('Ctrl Pts',(0.15681442133453,-0.190326085855194,-0.968453058988463));
#5206=CARTESIAN_POINT('Ctrl Pts',(0.139836317888042,-0.203463743702801,
-0.971100730005489));
#5207=CARTESIAN_POINT('Ctrl Pts',(0.104422493053067,-0.224161999508995,
-0.975530745318961));
#5208=CARTESIAN_POINT('Ctrl Pts',(0.0842175114474173,-0.232861760990032,
-0.977553872336861));
#5209=CARTESIAN_POINT('Ctrl Pts',(0.0421062857595698,-0.244251601209411,
-0.980270995488453));
#5210=CARTESIAN_POINT('Ctrl Pts',(0.0201990724523194,-0.246942143572133,
-0.980948));
#5211=CARTESIAN_POINT('Ctrl Pts',(-0.0201990724523193,-0.246942143572133,
-0.980948));
#5212=CARTESIAN_POINT('Ctrl Pts',(-0.0421062857595697,-0.244251601209411,
-0.980270995488453));
#5213=CARTESIAN_POINT('Ctrl Pts',(-0.0842175114474171,-0.232861760990032,
-0.977553872336861));
#5214=CARTESIAN_POINT('Ctrl Pts',(-0.104422493053067,-0.224161999508995,
-0.975530745318961));
#5215=CARTESIAN_POINT('Ctrl Pts',(-0.139836317888042,-0.203463743702801,
-0.971100730005489));
#5216=CARTESIAN_POINT('Ctrl Pts',(-0.15681442133453,-0.190326085855194,
-0.968453058988463));
#5217=CARTESIAN_POINT('Ctrl Pts',(-0.1868781821531,-0.15976606450048,-0.963103647174702));
#5218=CARTESIAN_POINT('Ctrl Pts',(-0.199966927975188,-0.142345102874864,
-0.960411259488514));
#5219=CARTESIAN_POINT('Ctrl Pts',(-0.223801617934945,-0.099930567888331,
-0.955173119738174));
#5220=CARTESIAN_POINT('Ctrl Pts',(-0.233157223576062,-0.0740444353928835,
-0.952850216871763));
#5221=CARTESIAN_POINT('Ctrl Pts',(-0.238183666596899,-0.0476299999999999,
-0.951592097314));
#5222=CARTESIAN_POINT('Origin',(5.55111512312578E-17,-0.04763,-1.));
#5223=CARTESIAN_POINT('Origin',(0.,-0.04763,0.));
#5224=CARTESIAN_POINT('',(0.504455939115715,-0.04763,-0.841298510752802));
#5225=CARTESIAN_POINT('Origin',(0.,-0.04763,0.));
#5226=CARTESIAN_POINT('Origin',(0.707106781186548,-0.04763,-0.707106781186547));
#5227=CARTESIAN_POINT('Origin',(0.707106781186548,0.,-0.707106781186547));
#5228=CARTESIAN_POINT('',(0.841298510752802,-0.04763,-0.504455939115715));
#5229=CARTESIAN_POINT('Ctrl Pts',(0.841298510752802,-0.04763,-0.504455939115715));
#5230=CARTESIAN_POINT('Ctrl Pts',(0.838633903678357,-0.0740444353928835,
-0.508899795931835));
#5231=CARTESIAN_POINT('Ctrl Pts',(0.833661031856294,-0.0999305678883309,
-0.517157748491652));
#5232=CARTESIAN_POINT('Ctrl Pts',(0.820511285096538,-0.142345102874864,
-0.537715343527944));
#5233=CARTESIAN_POINT('Ctrl Pts',(0.813159949759,-0.159766064500479,-0.548874290046456));
#5234=CARTESIAN_POINT('Ctrl Pts',(0.795684265985088,-0.190326085855194,
-0.573915184558107));
#5235=CARTESIAN_POINT('Ctrl Pts',(0.78555112003688,-0.203463743702801,-0.587792702767295));
#5236=CARTESIAN_POINT('Ctrl Pts',(0.763642258217233,-0.224161999508995,
-0.615966552324775));
#5237=CARTESIAN_POINT('Ctrl Pts',(0.750785745543687,-0.232861760990032,
-0.631684198665438));
#5238=CARTESIAN_POINT('Ctrl Pts',(0.722929908501543,-0.244251601209411,
-0.663382628119203));
#5239=CARTESIAN_POINT('Ctrl Pts',(0.707917883896095,-0.246942143572133,
-0.679352081686668));
#5240=CARTESIAN_POINT('Ctrl Pts',(0.679352081686668,-0.246942143572133,
-0.707917883896095));
#5241=CARTESIAN_POINT('Ctrl Pts',(0.663382628119203,-0.244251601209411,
-0.722929908501543));
#5242=CARTESIAN_POINT('Ctrl Pts',(0.631684198665438,-0.232861760990032,
-0.750785745543687));
#5243=CARTESIAN_POINT('Ctrl Pts',(0.615966552324775,-0.224161999508995,
-0.763642258217232));
#5244=CARTESIAN_POINT('Ctrl Pts',(0.587792702767295,-0.203463743702801,
-0.78555112003688));
#5245=CARTESIAN_POINT('Ctrl Pts',(0.573915184558107,-0.190326085855194,
-0.795684265985088));
#5246=CARTESIAN_POINT('Ctrl Pts',(0.548874290046456,-0.159766064500479,
-0.813159949759));
#5247=CARTESIAN_POINT('Ctrl Pts',(0.537715343527944,-0.142345102874864,
-0.820511285096538));
#5248=CARTESIAN_POINT('Ctrl Pts',(0.517157748491652,-0.099930567888331,
-0.833661031856294));
#5249=CARTESIAN_POINT('Ctrl Pts',(0.508899795931835,-0.0740444353928835,
-0.838633903678357));
#5250=CARTESIAN_POINT('Ctrl Pts',(0.504455939115715,-0.04763,-0.841298510752801));
#5251=CARTESIAN_POINT('Origin',(0.707106781186548,-0.04763,-0.707106781186547));
#5252=CARTESIAN_POINT('Origin',(0.,-0.166705,0.));
#5253=CARTESIAN_POINT('',(-0.980948,-0.28578,1.20131482833E-16));
#5254=CARTESIAN_POINT('Origin',(0.,-0.28578,0.));
#5255=CARTESIAN_POINT('',(-0.980948,-0.166705,1.20131482833E-16));
#5256=CARTESIAN_POINT('',(0.951592097314,-0.04763,0.238183666596899));
#5257=CARTESIAN_POINT('Origin',(0.,-0.04763,0.));
#5258=CARTESIAN_POINT('',(0.951592097314,-0.04763,-0.238183666596899));
#5259=CARTESIAN_POINT('Ctrl Pts',(0.951592097314,-0.04763,0.238183666596899));
#5260=CARTESIAN_POINT('Ctrl Pts',(0.952850216871763,-0.0740444353928835,
0.233157223576062));
#5261=CARTESIAN_POINT('Ctrl Pts',(0.955173119738174,-0.099930567888331,
0.223801617934945));
#5262=CARTESIAN_POINT('Ctrl Pts',(0.960411259488514,-0.142345102874864,
0.199966927975188));
#5263=CARTESIAN_POINT('Ctrl Pts',(0.963103647174702,-0.15976606450048,0.1868781821531));
#5264=CARTESIAN_POINT('Ctrl Pts',(0.968453058988463,-0.190326085855194,
0.15681442133453));
#5265=CARTESIAN_POINT('Ctrl Pts',(0.971100730005489,-0.203463743702801,
0.139836317888042));
#5266=CARTESIAN_POINT('Ctrl Pts',(0.975530745318961,-0.224161999508995,
0.104422493053067));
#5267=CARTESIAN_POINT('Ctrl Pts',(0.977553872336861,-0.232861760990032,
0.0842175114474172));
#5268=CARTESIAN_POINT('Ctrl Pts',(0.980270995488453,-0.244251601209411,
0.0421062857595697));
#5269=CARTESIAN_POINT('Ctrl Pts',(0.980948,-0.246942143572133,0.0201990724523194));
#5270=CARTESIAN_POINT('Ctrl Pts',(0.980948,-0.246942143572133,-0.0201990724523194));
#5271=CARTESIAN_POINT('Ctrl Pts',(0.980270995488453,-0.244251601209411,
-0.0421062857595697));
#5272=CARTESIAN_POINT('Ctrl Pts',(0.977553872336861,-0.232861760990032,
-0.0842175114474172));
#5273=CARTESIAN_POINT('Ctrl Pts',(0.975530745318961,-0.224161999508995,
-0.104422493053067));
#5274=CARTESIAN_POINT('Ctrl Pts',(0.971100730005489,-0.203463743702801,
-0.139836317888042));
#5275=CARTESIAN_POINT('Ctrl Pts',(0.968453058988463,-0.190326085855194,
-0.15681442133453));
#5276=CARTESIAN_POINT('Ctrl Pts',(0.963103647174702,-0.15976606450048,-0.1868781821531));
#5277=CARTESIAN_POINT('Ctrl Pts',(0.960411259488514,-0.142345102874864,
-0.199966927975188));
#5278=CARTESIAN_POINT('Ctrl Pts',(0.955173119738174,-0.099930567888331,
-0.223801617934945));
#5279=CARTESIAN_POINT('Ctrl Pts',(0.952850216871763,-0.0740444353928835,
-0.233157223576062));
#5280=CARTESIAN_POINT('Ctrl Pts',(0.951592097314,-0.0476299999999999,-0.238183666596899));
#5281=CARTESIAN_POINT('Origin',(0.,-0.04763,0.));
#5282=CARTESIAN_POINT('Origin',(0.,-0.04763,0.));
#5283=CARTESIAN_POINT('Origin',(1.,-0.04763,0.));
#5284=CARTESIAN_POINT('Origin',(1.,0.,0.));
#5285=CARTESIAN_POINT('Origin',(1.,-0.04763,0.));
#5286=CARTESIAN_POINT('Origin',(0.,-0.28578,0.));
#5287=CARTESIAN_POINT('Origin',(0.,-0.04763,0.));
#5355=UNCERTAINTY_MEASURE_WITH_UNIT(LENGTH_MEASURE(0.001),#5386,
'DISTANCE_ACCURACY_VALUE',
'Maximum model space distance between geometric entities at asserted c
onnectivities');
#5357=UNCERTAINTY_MEASURE_WITH_UNIT(LENGTH_MEASURE(0.001),#5386,
'DISTANCE_ACCURACY_VALUE',
'Maximum model space distance between geometric entities at asserted c
onnectivities');
#5383=(
GEOMETRIC_REPRESENTATION_CONTEXT(3)
GLOBAL_UNCERTAINTY_ASSIGNED_CONTEXT((#5355))
GLOBAL_UNIT_ASSIGNED_CONTEXT((#5386,#5388,#5389))
REPRESENTATION_CONTEXT('','3D')
);
#5385=(
GEOMETRIC_REPRESENTATION_CONTEXT(3)
GLOBAL_UNCERTAINTY_ASSIGNED_CONTEXT((#5357))
GLOBAL_UNIT_ASSIGNED_CONTEXT((#5386,#5388,#5389))
REPRESENTATION_CONTEXT('','3D')
);
#5386=(
LENGTH_UNIT()
NAMED_UNIT(*)
SI_UNIT(.CENTI.,.METRE.)
);
#5388=(
NAMED_UNIT(*)
PLANE_ANGLE_UNIT()
SI_UNIT($,.RADIAN.)
);
#5389=(
NAMED_UNIT(*)
SI_UNIT($,.STERADIAN.)
SOLID_ANGLE_UNIT()
);
#5415=SHAPE_DEFINITION_REPRESENTATION(#5456,#5496);
#5456=PRODUCT_DEFINITION_SHAPE('',$,#5524);
#5496=SHAPE_REPRESENTATION('',(#3220),#5383);
#5498=PRODUCT_DEFINITION_CONTEXT('part definition',#5581,'design');
#5524=PRODUCT_DEFINITION('Cage','Cage',#5551,#5498);
#5551=PRODUCT_DEFINITION_FORMATION('',$,#5608);
#5581=APPLICATION_CONTEXT(
'Core Data for Automotive Mechanical Design Process');
#5582=PRODUCT_CONTEXT('part definition',#5581,'mechanical');
#5608=PRODUCT('Cage','Cage','Cage',(#5582));
#5666=COLOUR_RGB('Grey',0.48,0.52,0.57);
#5667=FILL_AREA_STYLE_COLOUR('',#5666);
#5668=FILL_AREA_STYLE('',(#5667));
#5669=SURFACE_STYLE_FILL_AREA(#5668);
#5670=SURFACE_SIDE_STYLE('',(#5669));
#5671=SURFACE_STYLE_USAGE(.BOTH.,#5670);
#5672=PRESENTATION_STYLE_ASSIGNMENT((#5671));
ENDSEC;
END-ISO-10303-21;
